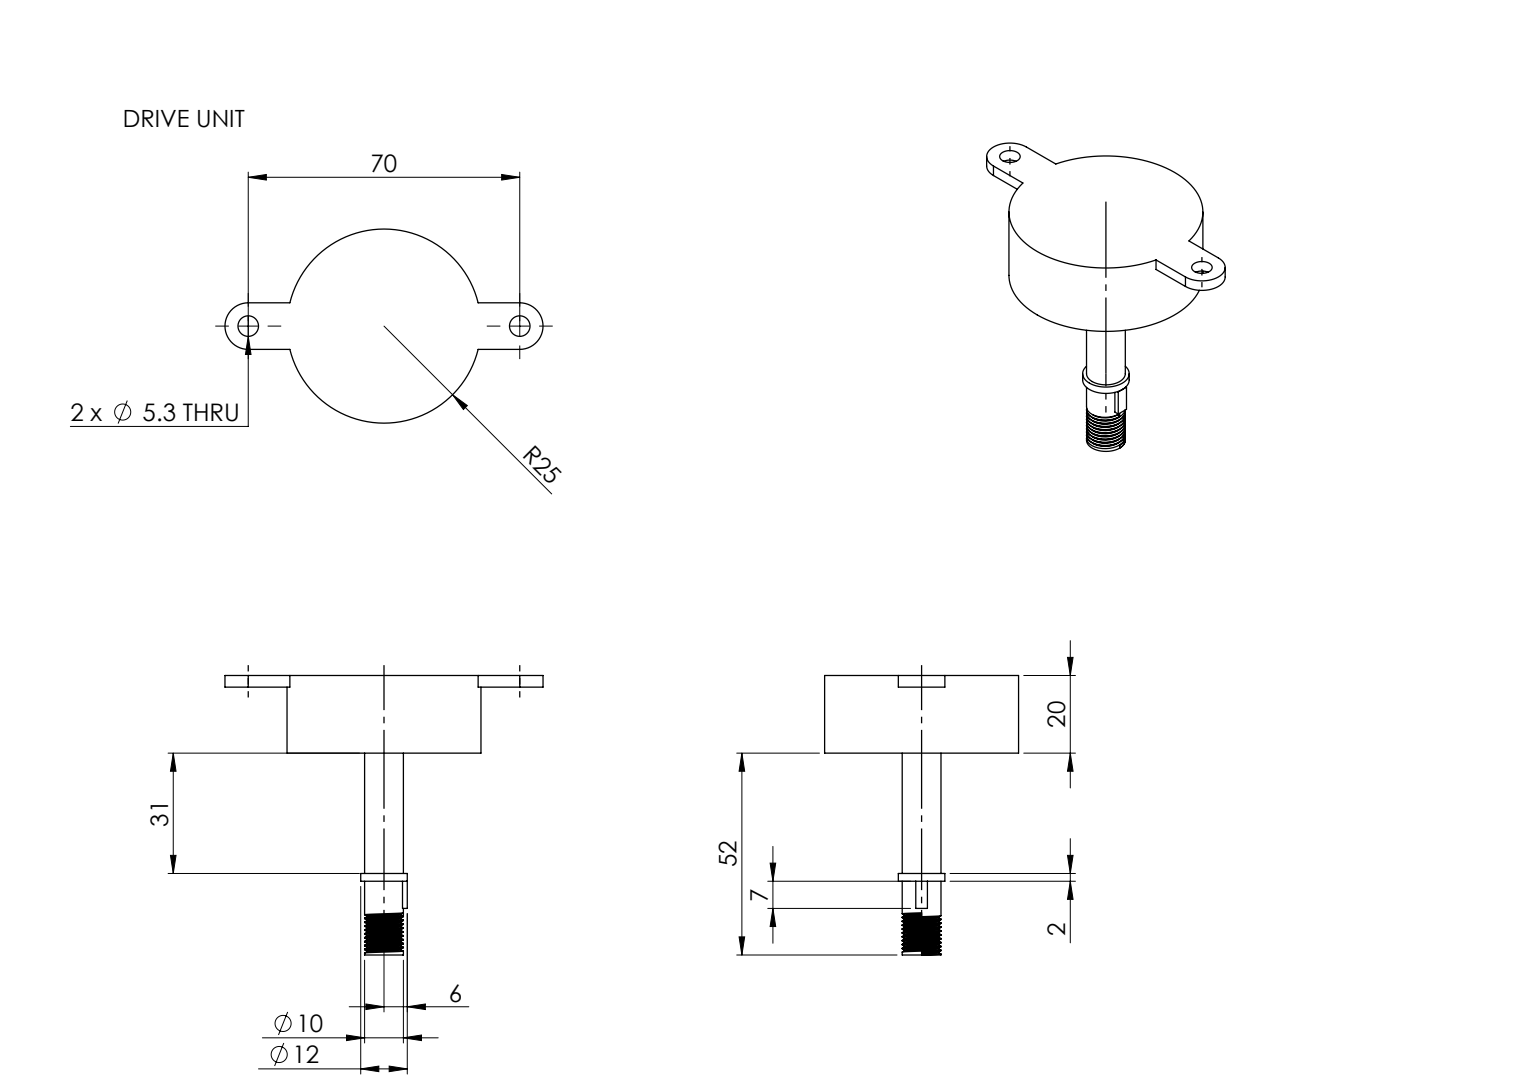
ISO-10303-21;
HEADER;
FILE_DESCRIPTION (('STEP AP214'),
    '1' );
FILE_NAME ('Drive Unit.step',
    '2026-10-08T13:56:24',
    ( '' ),
    ( '' ),
    'SwSTEP 2.0',
    'SolidWorks 2026',
    '' );
FILE_SCHEMA (( 'AUTOMOTIVE_DESIGN' ));
ENDSEC;

DATA;
#4=CARTESIAN_POINT ( 'NONE',  ( -1.846868145590737420, -24.75000000136559564, 4.458734124999999437 ) ) ;
#11=CARTESIAN_POINT ( 'NONE',  ( 1.846868145590735200, -25.50000000136559919, -4.458734125000000326 ) ) ;
#15=CARTESIAN_POINT ( 'NONE',  ( -3.535533905932738641, -28.50000000273118772, 3.535533905932737309 ) ) ;
#17=CARTESIAN_POINT ( 'NONE',  ( 3.152801135295367541, -29.31250000136559208, -3.152801135295367541 ) ) ;
#49=CARTESIAN_POINT ( 'NONE',  ( -2.071067811865478170, -24.31250000000000000, 5.000000000000000000 ) ) ;
#50=CARTESIAN_POINT ( 'NONE',  ( 5.000000000000000000, -28.18750000273119127, 2.071067811865478614 ) ) ;
#51=CARTESIAN_POINT ( 'NONE',  ( -4.458734124999999437, -26.25000000136559564, -1.846868145590735644 ) ) ;
#52=CARTESIAN_POINT ( 'NONE',  ( 3.152801135295366208, -23.56250000136559564, 3.152801135295367985 ) ) ;
#60=CARTESIAN_POINT ( 'NONE',  ( -4.458734124999999437, -23.18750000136559564, -5.460374474430324690E-16 ) ) ;
#62=CARTESIAN_POINT ( 'NONE',  ( -9.184850993605147944E-16, -30.37500000273118772, 5.000000000000000888 ) ) ;
#69=CARTESIAN_POINT ( 'NONE',  ( -3.535533905932737309, -27.62500000000000000, -3.535533905932738197 ) ) ;
#70=CARTESIAN_POINT ( 'NONE',  ( 1.846868145590736310, -28.62500000136559919, 4.458734124999999437 ) ) ;
#77=CARTESIAN_POINT ( 'NONE',  ( 2.730187237215162345E-16, -26.18750000136559564, -4.458734124999999437 ) ) ;
#79=VERTEX_POINT ( 'NONE', #13671 ) ;
#87=CARTESIAN_POINT ( 'NONE',  ( -3.535533905932738641, -30.37500000000000000, 3.535533905932737309 ) ) ;
#90=CARTESIAN_POINT ( 'NONE',  ( 3.535533905932738197, -27.00000000273118772, -3.535533905932738197 ) ) ;
#93=ORIENTED_EDGE ( 'NONE', *, *, #6840, .T. ) ;
#108=CARTESIAN_POINT ( 'NONE',  ( 5.000000000000000000, -24.06250000000000000, 2.071067811865478614 ) ) ;
#110=LINE ( 'NONE', #12615, #13102 ) ;
#113=FACE_OUTER_BOUND ( 'NONE', #15026, .T. ) ;
#122=DIRECTION ( 'NONE',  ( 0.000000000000000000, 0.000000000000000000, -1.000000000000000000 ) ) ;
#124=CARTESIAN_POINT ( 'NONE',  ( -9.184850993605147944E-16, -27.37500000273118772, 5.000000000000000000 ) ) ;
#129=CARTESIAN_POINT ( 'NONE',  ( 3.152801135295366208, -23.81250000136559564, 3.152801135295367985 ) ) ;
#130=ORIENTED_EDGE ( 'NONE', *, *, #2112, .F. ) ;
#136=EDGE_LOOP ( 'NONE', ( #1331, #8498 ) ) ;
#139=CARTESIAN_POINT ( 'NONE',  ( -1.846868145590737420, -25.00000000136559564, 4.458734124999999437 ) ) ;
#141=STYLED_ITEM ( 'NONE', ( #7237 ), #10261 ) ;
#143=PLANE ( 'NONE',  #15618 ) ;
#152=CARTESIAN_POINT ( 'NONE',  ( -1.846868145590734756, -25.12500000136559564, -4.458734125000000326 ) ) ;
#163=CARTESIAN_POINT ( 'NONE',  ( -4.458734124999999437, -25.93750000136559564, -5.460374474430324690E-16 ) ) ;
#164=ADVANCED_FACE ( 'NONE', ( #12534 ), #7474, .T. ) ;
#165=CARTESIAN_POINT ( 'NONE',  ( 0.000000000000000000, -13.00000000000000178, 0.000000000000000000 ) ) ;
#168=CARTESIAN_POINT ( 'NONE',  ( 6.123233995736766282E-16, -20.00000000000000000, -5.000000000000000000 ) ) ;
#172=CARTESIAN_POINT ( 'NONE',  ( 3.061616997868383141E-16, -30.75000000000000000, -5.000000000000000000 ) ) ;
#175=CARTESIAN_POINT ( 'NONE',  ( -3.535533905932738641, -27.50000000273118772, 3.535533905932737309 ) ) ;
#177=CARTESIAN_POINT ( 'NONE',  ( -1.846868145590734756, -31.12500000136559564, -4.458734124999999437 ) ) ;
#204=CARTESIAN_POINT ( 'NONE',  ( 1.846868145590735200, -31.25000000136559564, -4.458734125000000326 ) ) ;
#216=CARTESIAN_POINT ( 'NONE',  ( 3.061616997868383141E-16, -26.87500000273118772, -5.000000000000000000 ) ) ;
#217=CARTESIAN_POINT ( 'NONE',  ( 3.061616997868383141E-16, -27.87500000273118772, -5.000000000000000000 ) ) ;
#218=CARTESIAN_POINT ( 'NONE',  ( -1.846868145590737420, -22.00000000136559208, 4.458734124999997661 ) ) ;
#222=DIRECTION ( 'NONE',  ( -0.000000000000000000, 1.000000000000000000, -0.000000000000000000 ) ) ;
#227=EDGE_CURVE ( 'NONE', #9634, #14535, #13577, .T. ) ;
#228=ADVANCED_FACE ( 'NONE', ( #113 ), #1674, .T. ) ;
#234=CARTESIAN_POINT ( 'NONE',  ( 4.458734124999999437, -31.56250000136559564, 0.000000000000000000 ) ) ;
#240=CARTESIAN_POINT ( 'NONE',  ( 5.000000000000000000, -30.06250000000000000, 2.071067811865478614 ) ) ;
#243=CARTESIAN_POINT ( 'NONE',  ( -8.190561711645485556E-16, -26.68750000136559564, 4.458734124999999437 ) ) ;
#250=EDGE_CURVE ( 'NONE', #4014, #15267, #13743, .T. ) ;
#251=VECTOR ( 'NONE', #1802, 1000.000000000000000 ) ;
#252=CARTESIAN_POINT ( 'NONE',  ( -4.458734125000001214, -23.87500000136559564, 1.846868145590734089 ) ) ;
#257=DIRECTION ( 'NONE',  ( -0.000000000000000000, 1.000000000000000000, -0.000000000000000000 ) ) ;
#259=FACE_OUTER_BOUND ( 'NONE', #15924, .T. ) ;
#260=CARTESIAN_POINT ( 'NONE',  ( 5.000000000000000000, -29.00000000000000000, 0.000000000000000000 ) ) ;
#261=DIRECTION ( 'NONE',  ( -1.000000000000000000, 0.000000000000000000, 1.239088197126290570E-16 ) ) ;
#262=FACE_OUTER_BOUND ( 'NONE', #12296, .T. ) ;
#263=CARTESIAN_POINT ( 'NONE',  ( 2.071067811865476394, -27.31250000273118417, 5.000000000000000000 ) ) ;
#265=CARTESIAN_POINT ( 'NONE',  ( -8.190561711645485556E-16, -28.68750000136559564, 4.458734124999999437 ) ) ;
#270=ORIENTED_EDGE ( 'NONE', *, *, #4846, .T. ) ;
#274=CARTESIAN_POINT ( 'NONE',  ( 4.458734125000000326, -30.62500000136559208, -1.846868145590734978 ) ) ;
#278=( BOUNDED_CURVE ( )  B_SPLINE_CURVE ( 2, ( #14307, #13082, #15370, #11632, #13162, #12840, #4291, #11788, #15531 ),
 .UNSPECIFIED., .F., .F. ) 
 B_SPLINE_CURVE_WITH_KNOTS ( ( 3, 2, 2, 2, 3 ),
 ( 0.1750000000000001554, 0.1875000000000000833, 0.2000000000000000111, 0.2124999999999999389, 0.2249999999999998668 ),
 .UNSPECIFIED. ) 
 CURVE ( )  GEOMETRIC_REPRESENTATION_ITEM ( )  RATIONAL_B_SPLINE_CURVE ( ( 0.9999999999999990008, 0.9238795325112877377, 1.000000000000000000, 0.9238795325112867385, 1.000000000000000000, 0.9238795325112867385, 1.000000000000000000, 0.9238795325112876267, 0.9999999999999991118 ) ) 
 REPRESENTATION_ITEM ( '' )  );
#291=CARTESIAN_POINT ( 'NONE',  ( -9.184850993605147944E-16, -28.37500000273118772, 5.000000000000000000 ) ) ;
#292=EDGE_CURVE ( 'NONE', #10237, #3154, #5220, .T. ) ;
#293=CARTESIAN_POINT ( 'NONE',  ( -9.184850993605147944E-16, -21.37500000273118772, 5.000000000000000000 ) ) ;
#301=CYLINDRICAL_SURFACE ( 'NONE', #15098, 2.649999999999992806 ) ;
#305=CARTESIAN_POINT ( 'NONE',  ( -24.26932219902320043, 37.00000000000000000, -5.999999999999984901 ) ) ;
#308=ORIENTED_EDGE ( 'NONE', *, *, #7729, .F. ) ;
#311=DIRECTION ( 'NONE',  ( -0.000000000000000000, 1.000000000000000000, -0.000000000000000000 ) ) ;
#321=CARTESIAN_POINT ( 'NONE',  ( -3.152801135295367985, -22.81250000136559564, 3.152801135295367096 ) ) ;
#324=DIRECTION ( 'NONE',  ( 0.000000000000000000, 1.000000000000000000, 0.000000000000000000 ) ) ;
#328=CARTESIAN_POINT ( 'NONE',  ( 1.846868145590735200, -22.25000000136559564, -4.458734125000000326 ) ) ;
#331=CARTESIAN_POINT ( 'NONE',  ( -5.000000000000000888, -28.56250000000000000, -2.071067811865475949 ) ) ;
#335=EDGE_CURVE ( 'NONE', #10196, #14496, #7821, .T. ) ;
#336=CARTESIAN_POINT ( 'NONE',  ( -3.535533905932737309, -29.62500000000000355, -3.535533905932738197 ) ) ;
#339=CARTESIAN_POINT ( 'NONE',  ( 3.535533905932736864, -23.25000000273118772, 3.535533905932738641 ) ) ;
#341=CARTESIAN_POINT ( 'NONE',  ( -9.184850993605147944E-16, -24.37500000273118772, 5.000000000000000000 ) ) ;
#346=ORIENTED_EDGE ( 'NONE', *, *, #4980, .T. ) ;
#349=VERTEX_POINT ( 'NONE', #8867 ) ;
#351=CARTESIAN_POINT ( 'NONE',  ( -5.000000000000000000, -31.50000000000000000, -6.123233995736766282E-16 ) ) ;
#352=PLANE ( 'NONE',  #15206 ) ;
#353=VECTOR ( 'NONE', #2265, 1000.000000000000000 ) ;
#356=DIRECTION ( 'NONE',  ( 0.000000000000000000, 0.000000000000000000, 1.000000000000000000 ) ) ;
#357=ORIENTED_EDGE ( 'NONE', *, *, #14558, .T. ) ;
#365=CARTESIAN_POINT ( 'NONE',  ( 3.061616997868383043E-15, 20.00000000000000000, -25.00000000000000000 ) ) ;
#367=CARTESIAN_POINT ( 'NONE',  ( 6.123233995736766282E-16, -20.00000000000000000, -5.000000000000000000 ) ) ;
#372=CARTESIAN_POINT ( 'NONE',  ( 1.846868145590736310, -21.87500000136559208, 4.458734124999997661 ) ) ;
#376=CARTESIAN_POINT ( 'NONE',  ( -3.535533905932738641, -26.50000000273118772, 3.535533905932737309 ) ) ;
#379=VERTEX_POINT ( 'NONE', #1738 ) ;
#391=CARTESIAN_POINT ( 'NONE',  ( -4.458734125000001214, -22.87500000136559564, 1.846868145590734089 ) ) ;
#397=ORIENTED_EDGE ( 'NONE', *, *, #8592, .F. ) ;
#399=CARTESIAN_POINT ( 'NONE',  ( 3.152801135295367541, -31.56250000136559564, -3.152801135295367541 ) ) ;
#401=CARTESIAN_POINT ( 'NONE',  ( 0.000000000000000000, -32.00000000000000000, 0.000000000000000000 ) ) ;
#403=CIRCLE ( 'NONE', #1678, 25.00000000000000000 ) ;
#409=CARTESIAN_POINT ( 'NONE',  ( 5.000000000000000000, -29.06250000000000000, 2.071067811865478614 ) ) ;
#413=CARTESIAN_POINT ( 'NONE',  ( -3.535533905932738641, -24.50000000273118772, 3.535533905932737309 ) ) ;
#414=AXIS2_PLACEMENT_3D ( 'NONE', #3644, #8589, #5995 ) ;
#416=CARTESIAN_POINT ( 'NONE',  ( 4.458734124999999437, -26.37500000136559564, -1.846868145590734978 ) ) ;
#417=CARTESIAN_POINT ( 'NONE',  ( -35.00000000000000000, 40.00000000000000000, 0.000000000000000000 ) ) ;
#422=ADVANCED_FACE ( 'NONE', ( #15007 ), #3921, .T. ) ;
#426=CIRCLE ( 'NONE', #9451, 2.649999999999985700 ) ;
#428=CARTESIAN_POINT ( 'NONE',  ( 1.846868145590735200, -30.50000000136559919, -4.458734125000000326 ) ) ;
#432=CARTESIAN_POINT ( 'NONE',  ( 4.729367062499999719, -31.84375000068279959, 0.000000000000000000 ) ) ;
#436=CARTESIAN_POINT ( 'NONE',  ( -4.458734124999999437, -30.93750000136559564, -5.460374474430324690E-16 ) ) ;
#445=CARTESIAN_POINT ( 'NONE',  ( -3.535533905932737309, -28.75000000273118772, -3.535533905932738197 ) ) ;
#446=EDGE_CURVE ( 'NONE', #12836, #3368, #3237, .T. ) ;
#453=CARTESIAN_POINT ( 'NONE',  ( 3.152801135295367541, -23.56250000136559564, -3.152801135295367541 ) ) ;
#455=FACE_BOUND ( 'NONE', #11569, .T. ) ;
#464=( BOUNDED_CURVE ( )  B_SPLINE_CURVE ( 2, ( #5096, #12595, #1539, #6477, #12273, #177, #13559, #9939, #5254, #10191, #8585, #11390, #3640, #13806, #11315, #2658, #13474, #3714, #1368, #10032, #8661, #14967, #11084, #13650, #3882, #14877, #8901, #7611, #2741, #2411, #2579, #6158, #7531, #7454, #17, #4935, #12359, #12432, #15041, #1291, #8824, #12510, #6236, #11152, #265, #13725, #1451, #5010, #15363, #6792, #8985, #12990, #6636, #5424, #14147, #9068, #4372, #6553, #3076, #5661, #1695, #15207, #1612, #15451, #1927, #4120, #11550, #4034, #6877, #13898, #11468, #10427, #14227, #5497, #576, #7936, #12915, #7853, #11782, #4285, #12670, #416, #15113, #9305, #10278, #2826, #736, #7780, #4197, #11626, #3151, #9223, #8096, #8018, #11700, #1849, #504, #9144, #5339, #13970, #2902, #12750, #2984, #10356, #15283, #14057, #12833, #1777, #655, #5581, #6725, #10517, #810, #8263, #7406, #13156, #5730, #5809, #14834, #8701, #6110, #13603, #2090, #887, #9821, #4518, #52, #2013, #14750, #1328, #7035, #11935, #7323, #12310, #3600, #9453, #12227, #10665, #1249, #7489, #15600, #11037, #9895, #1166, #11027, #8547, #8620, #3311, #12392, #4896, #8175, #10601, #2451, #13435, #6197, #10745, #15525, #4968, #11114, #15681, #4441 ),
 .UNSPECIFIED., .F., .F. ) 
 B_SPLINE_CURVE_WITH_KNOTS ( ( 3, 2, 2, 2, 2, 2, 2, 2, 2, 2, 2, 2, 2, 2, 2, 2, 2, 2, 2, 2, 2, 2, 2, 2, 2, 2, 2, 2, 2, 2, 2, 2, 2, 2, 2, 2, 2, 2, 2, 2, 2, 2, 2, 2, 2, 2, 2, 2, 2, 2, 2, 2, 2, 2, 2, 2, 2, 2, 2, 2, 2, 2, 2, 2, 2, 2, 2, 2, 2, 2, 2, 2, 2, 2, 2, 2, 2, 2, 2, 2, 3 ),
 ( 0.000000000000000000, 0.01250000000000000069, 0.02500000000000000139, 0.03749999999999999861, 0.05000000000000000278, 0.06250000000000000000, 0.07499999999999999722, 0.08749999999999999445, 0.1000000000000000056, 0.1125000000000000028, 0.1250000000000000000, 0.1375000000000000111, 0.1499999999999999944, 0.1625000000000000056, 0.1749999999999999889, 0.1875000000000000000, 0.2000000000000000111, 0.2124999999999999944, 0.2250000000000000056, 0.2374999999999999889, 0.2500000000000000000, 0.2625000000000000111, 0.2750000000000000222, 0.2874999999999999778, 0.2999999999999999889, 0.3125000000000000000, 0.3250000000000000111, 0.3375000000000000222, 0.3499999999999999778, 0.3624999999999999889, 0.3750000000000000000, 0.3875000000000000111, 0.4000000000000000222, 0.4124999999999999778, 0.4249999999999999889, 0.4375000000000000000, 0.4500000000000000111, 0.4625000000000000222, 0.4749999999999999778, 0.4874999999999999889, 0.5000000000000000000, 0.5124999999999999556, 0.5250000000000000222, 0.5374999999999999778, 0.5500000000000000444, 0.5625000000000000000, 0.5749999999999999556, 0.5875000000000000222, 0.5999999999999999778, 0.6125000000000000444, 0.6250000000000000000, 0.6374999999999999556, 0.6500000000000000222, 0.6624999999999999778, 0.6750000000000000444, 0.6875000000000000000, 0.6999999999999999556, 0.7125000000000000222, 0.7249999999999999778, 0.7375000000000000444, 0.7500000000000000000, 0.7624999999999999556, 0.7750000000000000222, 0.7874999999999999778, 0.8000000000000000444, 0.8125000000000000000, 0.8249999999999999556, 0.8375000000000000222, 0.8499999999999999778, 0.8625000000000000444, 0.8750000000000000000, 0.8874999999999999556, 0.9000000000000000222, 0.9124999999999999778, 0.9250000000000000444, 0.9375000000000000000, 0.9499999999999999556, 0.9625000000000000222, 0.9749999999999999778, 0.9875000000000000444, 1.000000000000000000 ),
 .UNSPECIFIED. ) 
 CURVE ( )  GEOMETRIC_REPRESENTATION_ITEM ( )  RATIONAL_B_SPLINE_CURVE ( ( 1.000000000000000000, 0.9238795325112867385, 1.000000000000000000, 0.9238795325112867385, 1.000000000000000000, 0.9238795325112867385, 1.000000000000000000, 0.9238795325112867385, 1.000000000000000000, 0.9238795325112867385, 1.000000000000000000, 0.9238795325112867385, 1.000000000000000000, 0.9238795325112867385, 1.000000000000000000, 0.9238795325112867385, 1.000000000000000000, 0.9238795325112867385, 1.000000000000000000, 0.9238795325112867385, 1.000000000000000000, 0.9238795325112867385, 1.000000000000000000, 0.9238795325112867385, 1.000000000000000000, 0.9238795325112867385, 1.000000000000000000, 0.9238795325112867385, 1.000000000000000000, 0.9238795325112867385, 1.000000000000000000, 0.9238795325112867385, 1.000000000000000000, 0.9238795325112867385, 1.000000000000000000, 0.9238795325112867385, 1.000000000000000000, 0.9238795325112867385, 1.000000000000000000, 0.9238795325112867385, 1.000000000000000000, 0.9238795325112867385, 1.000000000000000000, 0.9238795325112867385, 1.000000000000000000, 0.9238795325112867385, 1.000000000000000000, 0.9238795325112867385, 1.000000000000000000, 0.9238795325112867385, 1.000000000000000000, 0.9238795325112867385, 1.000000000000000000, 0.9238795325112867385, 1.000000000000000000, 0.9238795325112867385, 1.000000000000000000, 0.9238795325112867385, 1.000000000000000000, 0.9238795325112867385, 1.000000000000000000, 0.9238795325112867385, 1.000000000000000000, 0.9238795325112867385, 1.000000000000000000, 0.9238795325112867385, 1.000000000000000000, 0.9238795325112867385, 1.000000000000000000, 0.9238795325112867385, 1.000000000000000000, 0.9238795325112867385, 1.000000000000000000, 0.9238795325112867385, 1.000000000000000000, 0.9238795325112867385, 1.000000000000000000, 0.9238795325112867385, 1.000000000000000000, 0.9238795325112867385, 1.000000000000000000, 0.9238795325112867385, 1.000000000000000000, 0.9238795325112867385, 1.000000000000000000, 0.9238795325112867385, 1.000000000000000000, 0.9238795325112867385, 1.000000000000000000, 0.9238795325112867385, 1.000000000000000000, 0.9238795325112867385, 1.000000000000000000, 0.9238795325112867385, 1.000000000000000000, 0.9238795325112867385, 1.000000000000000000, 0.9238795325112867385, 1.000000000000000000, 0.9238795325112867385, 1.000000000000000000, 0.9238795325112867385, 1.000000000000000000, 0.9238795325112867385, 1.000000000000000000, 0.9238795325112867385, 1.000000000000000000, 0.9238795325112867385, 1.000000000000000000, 0.9238795325112867385, 1.000000000000000000, 0.9238795325112867385, 1.000000000000000000, 0.9238795325112867385, 1.000000000000000000, 0.9238795325112867385, 1.000000000000000000, 0.9238795325112867385, 1.000000000000000000, 0.9238795325112867385, 1.000000000000000000, 0.9238795325112867385, 1.000000000000000000, 0.9238795325112867385, 1.000000000000000000, 0.9238795325112867385, 1.000000000000000000, 0.9238795325112867385, 1.000000000000000000, 0.9238795325112867385, 1.000000000000000000, 0.9238795325112867385, 1.000000000000000000, 0.9238795325112867385, 1.000000000000000000, 0.9238795325112867385, 1.000000000000000000, 0.9238795325112867385, 1.000000000000000000, 0.9238795325112867385, 1.000000000000000000, 0.9238795325112867385, 1.000000000000000000, 0.9238795325112867385, 1.000000000000000000, 0.9238795325112867385, 1.000000000000000000, 0.9238795325112867385, 1.000000000000000000, 0.9238795325112867385, 1.000000000000000000, 0.9238795325112867385, 1.000000000000000000, 0.9238795325112867385, 1.000000000000000000, 0.9238795325112867385, 1.000000000000000000, 0.9238795325112867385, 1.000000000000000000, 0.9238795325112867385, 1.000000000000000000 ) ) 
 REPRESENTATION_ITEM ( '' )  );
#469=FACE_OUTER_BOUND ( 'NONE', #10752, .T. ) ;
#476=CARTESIAN_POINT ( 'NONE',  ( 1.846868145590735200, -24.25000000136559564, -4.458734125000000326 ) ) ;
#479=UNCERTAINTY_MEASURE_WITH_UNIT (LENGTH_MEASURE( 1.000000000000000082E-05 ), #11657, 'distance_accuracy_value', 'NONE');
#481=DIRECTION ( 'NONE',  ( 0.000000000000000000, 0.000000000000000000, 1.000000000000000000 ) ) ;
#483=ORIENTED_EDGE ( 'NONE', *, *, #15732, .F. ) ;
#484=ORIENTED_EDGE ( 'NONE', *, *, #9626, .T. ) ;
#485=CARTESIAN_POINT ( 'NONE',  ( 1.846868145590736310, -21.62500000136559564, 4.458734124999999437 ) ) ;
#488=DIRECTION ( 'NONE',  ( 0.000000000000000000, -0.000000000000000000, 1.000000000000000000 ) ) ;
#491=DIRECTION ( 'NONE',  ( 0.000000000000000000, 1.000000000000000000, 0.000000000000000000 ) ) ;
#494=CARTESIAN_POINT ( 'NONE',  ( 2.071067811865476394, -26.18750000000000355, 5.000000000000000000 ) ) ;
#499=EDGE_CURVE ( 'NONE', #2433, #13770, #15943, .T. ) ;
#500=CARTESIAN_POINT ( 'NONE',  ( -2.071067811865475061, -24.81250000273118417, -5.000000000000000888 ) ) ;
#503=CIRCLE ( 'NONE', #4355, 5.000000000000000000 ) ;
#504=CARTESIAN_POINT ( 'NONE',  ( 4.458734124999999437, -25.43750000136559564, 0.000000000000000000 ) ) ;
#517=DIRECTION ( 'NONE',  ( 1.000000000000000000, -0.000000000000000000, -1.239088197126290570E-16 ) ) ;
#521=EDGE_CURVE ( 'NONE', #13476, #13669, #12188, .T. ) ;
#528=CARTESIAN_POINT ( 'NONE',  ( -4.458734125000001214, -27.87500000136559564, 1.846868145590734089 ) ) ;
#529=ORIENTED_EDGE ( 'NONE', *, *, #6898, .T. ) ;
#538=CARTESIAN_POINT ( 'NONE',  ( -4.458734124999999437, -23.18750000136559564, -5.460374474430324690E-16 ) ) ;
#539=ORIENTED_EDGE ( 'NONE', *, *, #227, .F. ) ;
#548=CARTESIAN_POINT ( 'NONE',  ( 0.000000000000000000, -20.00000000000000000, 0.000000000000000000 ) ) ;
#552=CARTESIAN_POINT ( 'NONE',  ( 5.000000000000000000, -23.06250000000000000, 2.071067811865478614 ) ) ;
#555=CARTESIAN_POINT ( 'NONE',  ( 5.000000000000000888, -25.06250000273118417, -2.071067811865475505 ) ) ;
#556=FACE_OUTER_BOUND ( 'NONE', #7798, .T. ) ;
#562=CARTESIAN_POINT ( 'NONE',  ( 1.846868145590736310, -30.87500000136559564, 4.458734124999999437 ) ) ;
#570=CARTESIAN_POINT ( 'NONE',  ( -5.000000000000000000, -27.50000000000000000, -6.123233995736766282E-16 ) ) ;
#574=CARTESIAN_POINT ( 'NONE',  ( 5.000000000000000000, -23.18750000273119127, 2.071067811865478614 ) ) ;
#576=CARTESIAN_POINT ( 'NONE',  ( -3.152801135295367985, -26.81250000136559564, 3.152801135295367096 ) ) ;
#580=VERTEX_POINT ( 'NONE', #7452 ) ;
#583=ORIENTED_EDGE ( 'NONE', *, *, #907, .F. ) ;
#588=CARTESIAN_POINT ( 'NONE',  ( -3.152801135295367985, -26.06250000136559919, 3.152801135295367096 ) ) ;
#594=EDGE_LOOP ( 'NONE', ( #1579, #15115, #2346, #7475 ) ) ;
#601=EDGE_CURVE ( 'NONE', #3228, #2810, #2578, .T. ) ;
#603=DIRECTION ( 'NONE',  ( -1.000000000000000000, 0.000000000000000000, 1.239088197126290570E-16 ) ) ;
#607=UNCERTAINTY_MEASURE_WITH_UNIT (LENGTH_MEASURE( 1.000000000000000082E-05 ), #5032, 'distance_accuracy_value', 'NONE');
#611=VECTOR ( 'NONE', #13383, 1000.000000000000000 ) ;
#614=CARTESIAN_POINT ( 'NONE',  ( 3.061616997868383141E-16, -24.75000000000000000, -5.000000000000000000 ) ) ;
#627=CARTESIAN_POINT ( 'NONE',  ( 5.000000000000000888, -26.06250000273118417, -2.071067811865475505 ) ) ;
#633=CARTESIAN_POINT ( 'NONE',  ( -3.152801135295367985, -21.81250000136559208, 3.152801135295367096 ) ) ;
#639=CARTESIAN_POINT ( 'NONE',  ( -4.458734125000000326, -22.00000000136559208, -1.846868145590735644 ) ) ;
#649=CARTESIAN_POINT ( 'NONE',  ( 5.000000000000000888, -27.93750000000000711, -2.071067811865475505 ) ) ;
#653=CARTESIAN_POINT ( 'NONE',  ( -9.184850993605147944E-16, -23.37500000273118772, 5.000000000000000000 ) ) ;
#654=ORIENTED_EDGE ( 'NONE', *, *, #7999, .T. ) ;
#655=CARTESIAN_POINT ( 'NONE',  ( -8.190561711645485556E-16, -24.68750000136559564, 4.458734124999999437 ) ) ;
#661=CARTESIAN_POINT ( 'NONE',  ( 4.769696007084728073, -20.00000000000000000, 1.500000000000000000 ) ) ;
#666=CARTESIAN_POINT ( 'NONE',  ( 3.152801135295367541, -26.56250000136559564, -3.152801135295367541 ) ) ;
#680=DIRECTION ( 'NONE',  ( -0.000000000000000000, -1.000000000000000000, -0.000000000000000000 ) ) ;
#689=EDGE_LOOP ( 'NONE', ( #8517, #6406, #1835, #397 ) ) ;
#693=CARTESIAN_POINT ( 'NONE',  ( 3.535533905932736864, -27.12500000000000000, 3.535533905932738641 ) ) ;
#695=ORIENTED_EDGE ( 'NONE', *, *, #15597, .F. ) ;
#704=CARTESIAN_POINT ( 'NONE',  ( -5.000000000000000000, -25.50000000000000355, -6.123233995736766282E-16 ) ) ;
#711=CARTESIAN_POINT ( 'NONE',  ( -4.458734124999999437, -28.25000000136559919, -1.846868145590735644 ) ) ;
#713=EDGE_CURVE ( 'NONE', #79, #15920, #10355, .T. ) ;
#719=CARTESIAN_POINT ( 'NONE',  ( -4.458734125000000326, -28.25000000136559208, -1.846868145590735644 ) ) ;
#720=CARTESIAN_POINT ( 'NONE',  ( 6.123233995736766282E-16, -20.00000000000000000, -5.000000000000000000 ) ) ;
#721=VECTOR ( 'NONE', #9973, 1000.000000000000114 ) ;
#727=DIRECTION ( 'NONE',  ( -0.000000000000000000, -1.000000000000000000, -0.000000000000000000 ) ) ;
#728=CARTESIAN_POINT ( 'NONE',  ( 5.000000000000000000, -24.00000000000000000, 0.000000000000000000 ) ) ;
#733=CARTESIAN_POINT ( 'NONE',  ( 5.000000000000000000, -21.18750000273119127, 2.071067811865478614 ) ) ;
#735=ORIENTED_EDGE ( 'NONE', *, *, #13938, .F. ) ;
#736=CARTESIAN_POINT ( 'NONE',  ( -3.152801135295367096, -26.06250000136559564, -3.152801135295367541 ) ) ;
#741=AXIS2_PLACEMENT_3D ( 'NONE', #14902, #12451, #7471 ) ;
#747=CARTESIAN_POINT ( 'NONE',  ( -1.846868145590734756, -29.37500000136559564, -4.458734125000000326 ) ) ;
#755=ORIENTED_EDGE ( 'NONE', *, *, #9626, .F. ) ;
#774=CARTESIAN_POINT ( 'NONE',  ( 5.000000000000000000, -27.00000000000000000, 0.000000000000000000 ) ) ;
#776=ORIENTED_EDGE ( 'NONE', *, *, #7729, .T. ) ;
#787=CARTESIAN_POINT ( 'NONE',  ( 3.061616997868383141E-16, -24.87500000273118417, -5.000000000000000000 ) ) ;
#788=CARTESIAN_POINT ( 'NONE',  ( 4.458734124999999437, -28.62500000136559564, -1.846868145590734978 ) ) ;
#796=CARTESIAN_POINT ( 'NONE',  ( 3.152801135295366208, -25.81250000136559564, 3.152801135295367985 ) ) ;
#804=CARTESIAN_POINT ( 'NONE',  ( -3.535533905932738641, -26.37500000000000355, 3.535533905932737309 ) ) ;
#808=CARTESIAN_POINT ( 'NONE',  ( -3.152801135295367096, -29.06250000136559564, -3.152801135295367541 ) ) ;
#809=ORIENTED_EDGE ( 'NONE', *, *, #11477, .T. ) ;
#810=CARTESIAN_POINT ( 'NONE',  ( 4.458734124999999437, -24.43750000136559564, 0.000000000000000000 ) ) ;
#813=ORIENTED_EDGE ( 'NONE', *, *, #12222, .F. ) ;
#815=CARTESIAN_POINT ( 'NONE',  ( -3.152801135295367096, -28.06250000136559564, -3.152801135295367541 ) ) ;
#818=CARTESIAN_POINT ( 'NONE',  ( -3.535533905932738641, -24.50000000273118772, 3.535533905932737309 ) ) ;
#821=CARTESIAN_POINT ( 'NONE',  ( -3.152801135295367096, -26.31250000136559564, -3.152801135295367541 ) ) ;
#822=DIRECTION ( 'NONE',  ( -1.000000000000000000, 0.000000000000000000, 1.239088197126290570E-16 ) ) ;
#829=EDGE_LOOP ( 'NONE', ( #13631, #3584, #12937, #6136 ) ) ;
#831=ORIENTED_EDGE ( 'NONE', *, *, #10965, .F. ) ;
#836=CARTESIAN_POINT ( 'NONE',  ( 3.061616997868383141E-16, -27.75000000000000000, -5.000000000000000000 ) ) ;
#846=EDGE_CURVE ( 'NONE', #8138, #15819, #13214, .T. ) ;
#851=EDGE_LOOP ( 'NONE', ( #9621, #3536, #2832, #14469 ) ) ;
#856=LINE ( 'NONE', #14435, #15169 ) ;
#858=CYLINDRICAL_SURFACE ( 'NONE', #8255, 5.000000000000000000 ) ;
#863=CARTESIAN_POINT ( 'NONE',  ( 1.846868145590736310, -27.87500000136559564, 4.458734124999997661 ) ) ;
#870=ADVANCED_FACE ( 'NONE', ( #1789 ), #9154, .T. ) ;
#875=CARTESIAN_POINT ( 'NONE',  ( 1.846868145590735200, -25.50000000136559919, -4.458734125000000326 ) ) ;
#880=( BOUNDED_CURVE ( )  B_SPLINE_CURVE ( 2, ( #1973, #6919, #693, #11825, #774, #5696, #10633, #15564, #1149 ),
 .UNSPECIFIED., .F., .F. ) 
 B_SPLINE_CURVE_WITH_KNOTS ( ( 3, 2, 2, 2, 3 ),
 ( 0.4750000000000000888, 0.4875000000000000999, 0.5000000000000001110, 0.5125000000000000666, 0.5250000000000001332 ),
 .UNSPECIFIED. ) 
 CURVE ( )  GEOMETRIC_REPRESENTATION_ITEM ( )  RATIONAL_B_SPLINE_CURVE ( ( 0.9999999999999993339, 0.9238795325112874046, 1.000000000000000000, 0.9238795325112867385, 1.000000000000000000, 0.9238795325112867385, 1.000000000000000000, 0.9238795325112860723, 1.000000000000000666 ) ) 
 REPRESENTATION_ITEM ( '' )  );
#885=CARTESIAN_POINT ( 'NONE',  ( 1.846868145590736310, -29.62500000136559208, 4.458734124999999437 ) ) ;
#887=CARTESIAN_POINT ( 'NONE',  ( -1.846868145590737420, -23.75000000136559564, 4.458734124999997661 ) ) ;
#895=CARTESIAN_POINT ( 'NONE',  ( -4.458734124999999437, -29.93750000136559564, -5.460374474430324690E-16 ) ) ;
#898=CARTESIAN_POINT ( 'NONE',  ( -5.000000000000000888, -24.56250000273118772, 2.071067811865474617 ) ) ;
#899=FACE_OUTER_BOUND ( 'NONE', #14701, .T. ) ;
#901=CARTESIAN_POINT ( 'NONE',  ( -8.190561711645485556E-16, -28.93750000136559564, 4.458734124999999437 ) ) ;
#907=EDGE_CURVE ( 'NONE', #8217, #4663, #4887, .T. ) ;
#909=ORIENTED_EDGE ( 'NONE', *, *, #7781, .F. ) ;
#926=AXIS2_PLACEMENT_3D ( 'NONE', #14707, #3629, #488 ) ;
#929=CARTESIAN_POINT ( 'NONE',  ( 6.000000000000000000, -13.00000000000000178, 1.500000000000000000 ) ) ;
#933=CIRCLE ( 'NONE', #2729, 5.000000000000000000 ) ;
#936=DIRECTION ( 'NONE',  ( 0.000000000000000000, 0.000000000000000000, -1.000000000000000000 ) ) ;
#940=CARTESIAN_POINT ( 'NONE',  ( -8.190561711645485556E-16, -30.93750000136559564, 4.458734124999999437 ) ) ;
#943=AXIS2_PLACEMENT_3D ( 'NONE', #9492, #14262, #5694 ) ;
#949=AXIS2_PLACEMENT_3D ( 'NONE', #12692, #12456, #11172 ) ;
#950=CARTESIAN_POINT ( 'NONE',  ( -8.190561711645485556E-16, -26.93750000136559564, 4.458734124999999437 ) ) ;
#951=DIRECTION ( 'NONE',  ( 0.000000000000000000, 0.000000000000000000, 1.000000000000000000 ) ) ;
#959=CARTESIAN_POINT ( 'NONE',  ( 5.000000000000000000, -23.06250000000000000, 2.071067811865478614 ) ) ;
#961=CARTESIAN_POINT ( 'NONE',  ( -5.000000000000000000, -21.62500000273118772, -6.123233995736766282E-16 ) ) ;
#962=CARTESIAN_POINT ( 'NONE',  ( 3.061616997868383141E-16, -27.75000000000000000, -5.000000000000000000 ) ) ;
#963=CARTESIAN_POINT ( 'NONE',  ( -9.184850993605147944E-16, -22.37500000273118417, 5.000000000000000000 ) ) ;
#970=CARTESIAN_POINT ( 'NONE',  ( -8.190561711645485556E-16, -28.68750000136559564, 4.458734124999999437 ) ) ;
#973=CARTESIAN_POINT ( 'NONE',  ( -2.071067811865492381, -24.43750000273118772, 4.999999999999985789 ) ) ;
#974=( BOUNDED_CURVE ( )  B_SPLINE_CURVE ( 2, ( #5596, #5515, #12932, #4387, #6567 ),
 .UNSPECIFIED., .F., .F. ) 
 B_SPLINE_CURVE_WITH_KNOTS ( ( 3, 2, 3 ),
 ( 0.000000000000000000, 0.01250000000000001110, 0.02500000000000002220 ),
 .UNSPECIFIED. ) 
 CURVE ( )  GEOMETRIC_REPRESENTATION_ITEM ( )  RATIONAL_B_SPLINE_CURVE ( ( 1.000000000000000000, 0.9238795325112867385, 1.000000000000000000, 0.9238795325112866275, 1.000000000000000222 ) ) 
 REPRESENTATION_ITEM ( '' )  );
#980=CARTESIAN_POINT ( 'NONE',  ( -1.846868145590734756, -23.37500000136559564, -4.458734125000000326 ) ) ;
#983=CARTESIAN_POINT ( 'NONE',  ( -2.071067811865475061, -30.81250000273118772, -5.000000000000000888 ) ) ;
#985=ORIENTED_EDGE ( 'NONE', *, *, #11874, .T. ) ;
#990=AXIS2_PLACEMENT_3D ( 'NONE', #10557, #15485, #3024 ) ;
#1004=ORIENTED_EDGE ( 'NONE', *, *, #13938, .T. ) ;
#1006=EDGE_LOOP ( 'NONE', ( #7439, #10537, #3336, #10117, #9918, #9746, #14886, #3496 ) ) ;
#1017=DIRECTION ( 'NONE',  ( 0.000000000000000000, 1.000000000000000000, 0.000000000000000000 ) ) ;
#1018=CARTESIAN_POINT ( 'NONE',  ( -3.152801135295367985, -29.06250000136559564, 3.152801135295367096 ) ) ;
#1026=CARTESIAN_POINT ( 'NONE',  ( -1.846868145590734756, -23.37500000136559564, -4.458734125000000326 ) ) ;
#1027=CARTESIAN_POINT ( 'NONE',  ( -35.00000000000000000, 37.00000000000000000, 0.000000000000000000 ) ) ;
#1035=CARTESIAN_POINT ( 'NONE',  ( 5.000000000000000888, -22.06250000273119127, -2.071067811865475505 ) ) ;
#1042=CARTESIAN_POINT ( 'NONE',  ( -3.152801135295367096, -29.06250000136559564, -3.152801135295367541 ) ) ;
#1043=EDGE_CURVE ( 'NONE', #8138, #8374, #4686, .T. ) ;
#1050=CARTESIAN_POINT ( 'NONE',  ( -1.846868145590734756, -22.37500000136559564, -4.458734125000000326 ) ) ;
#1053=CARTESIAN_POINT ( 'NONE',  ( -5.000000000000000888, -30.68750000273118772, -2.071067811865475949 ) ) ;
#1073=ORIENTED_EDGE ( 'NONE', *, *, #9578, .F. ) ;
#1086=CARTESIAN_POINT ( 'NONE',  ( -5.000000000000000000, -24.50000000000000000, -6.123233995736766282E-16 ) ) ;
#1088=CARTESIAN_POINT ( 'NONE',  ( 3.152801135295367541, -26.56250000136559564, -3.152801135295367541 ) ) ;
#1096=CARTESIAN_POINT ( 'NONE',  ( -3.152801135295367096, -23.31250000136559564, -3.152801135295367541 ) ) ;
#1097=DIRECTION ( 'NONE',  ( -0.000000000000000000, -1.000000000000000000, -0.000000000000000000 ) ) ;
#1100=DIRECTION ( 'NONE',  ( 0.000000000000000000, -1.000000000000000000, 0.000000000000000000 ) ) ;
#1102=CARTESIAN_POINT ( 'NONE',  ( 3.061616997868383141E-16, -23.75000000000000000, -5.000000000000000000 ) ) ;
#1105=LINE ( 'NONE', #10970, #4851 ) ;
#1106=CARTESIAN_POINT ( 'NONE',  ( -4.458734124999999437, -26.93750000136559564, -5.460374474430324690E-16 ) ) ;
#1108=VERTEX_POINT ( 'NONE', #2026 ) ;
#1111=ORIENTED_EDGE ( 'NONE', *, *, #5804, .F. ) ;
#1115=CARTESIAN_POINT ( 'NONE',  ( -4.458734125000001214, -24.87500000136559919, 1.846868145590734089 ) ) ;
#1123=CARTESIAN_POINT ( 'NONE',  ( -3.152801135295367096, -25.31250000136559564, -3.152801135295367541 ) ) ;
#1139=FACE_OUTER_BOUND ( 'NONE', #10434, .T. ) ;
#1140=EDGE_CURVE ( 'NONE', #4136, #11992, #9616, .T. ) ;
#1141=CARTESIAN_POINT ( 'NONE',  ( 3.535533905932738197, -27.87500000000000000, -3.535533905932738197 ) ) ;
#1149=CARTESIAN_POINT ( 'NONE',  ( 3.061616997868383141E-16, -26.75000000000000000, -5.000000000000000000 ) ) ;
#1162=CARTESIAN_POINT ( 'NONE',  ( -5.000000000000000888, -29.68750000273118417, -2.071067811865475949 ) ) ;
#1165=CARTESIAN_POINT ( 'NONE',  ( -8.190561711645485556E-16, -25.93750000136559564, 4.458734124999999437 ) ) ;
#1166=CARTESIAN_POINT ( 'NONE',  ( 4.458734124999997661, -22.50000000136559564, 1.846868145590737864 ) ) ;
#1172=ORIENTED_EDGE ( 'NONE', *, *, #6097, .F. ) ;
#1173=CARTESIAN_POINT ( 'NONE',  ( -3.152801135295367985, -25.06250000136559564, 3.152801135295367096 ) ) ;
#1174=CARTESIAN_POINT ( 'NONE',  ( -5.000000000000000000, -23.62500000273118772, -6.123233995736766282E-16 ) ) ;
#1177=CARTESIAN_POINT ( 'NONE',  ( 35.00000000000000000, 37.00000000000000000, 5.999999999999991118 ) ) ;
#1179=EDGE_CURVE ( 'NONE', #12690, #11826, #3166, .T. ) ;
#1187=CARTESIAN_POINT ( 'NONE',  ( 4.458734125000000326, -26.37500000136559564, -1.846868145590734978 ) ) ;
#1195=DIRECTION ( 'NONE',  ( -1.000000000000000000, 0.000000000000000000, -0.000000000000000000 ) ) ;
#1196=CARTESIAN_POINT ( 'NONE',  ( -1.846868145590737420, -23.75000000136559208, 4.458734124999999437 ) ) ;
#1204=CARTESIAN_POINT ( 'NONE',  ( 6.000000000000000000, -20.00000000000000000, 1.500000000000000000 ) ) ;
#1207=CARTESIAN_POINT ( 'NONE',  ( 2.730187237215162345E-16, -25.43750000136559564, -4.458734124999999437 ) ) ;
#1211=CARTESIAN_POINT ( 'NONE',  ( -5.000000000000000888, -28.68750000273119127, -2.071067811865475949 ) ) ;
#1219=CIRCLE ( 'NONE', #5862, 5.000000000000000000 ) ;
#1237=FACE_OUTER_BOUND ( 'NONE', #12435, .T. ) ;
#1243=CARTESIAN_POINT ( 'NONE',  ( 5.000000000000000000, -27.18750000273119127, 2.071067811865478614 ) ) ;
#1248=CARTESIAN_POINT ( 'NONE',  ( -1.846868145590734756, -27.37500000136559564, -4.458734124999999437 ) ) ;
#1249=CARTESIAN_POINT ( 'NONE',  ( -3.152801135295367985, -22.81250000136559564, 3.152801135295367096 ) ) ;
#1258=CARTESIAN_POINT ( 'NONE',  ( -8.190561711645485556E-16, -21.93750000136559208, 4.458734124999999437 ) ) ;
#1264=LINE ( 'NONE', #1177, #4309 ) ;
#1266=CIRCLE ( 'NONE', #10326, 5.000000000000000000 ) ;
#1270=CARTESIAN_POINT ( 'NONE',  ( 3.152801135295367541, -26.31250000136559564, -3.152801135295367541 ) ) ;
#1277=CARTESIAN_POINT ( 'NONE',  ( 1.846868145590735200, -25.25000000136559564, -4.458734125000000326 ) ) ;
#1286=CARTESIAN_POINT ( 'NONE',  ( 1.846868145590735200, -24.50000000136559564, -4.458734125000000326 ) ) ;
#1289=CARTESIAN_POINT ( 'NONE',  ( 3.535533905932738197, -28.00000000273118772, -3.535533905932738197 ) ) ;
#1291=CARTESIAN_POINT ( 'NONE',  ( -4.458734124999999437, -29.00000000136559564, -1.846868145590735644 ) ) ;
#1294=( BOUNDED_CURVE ( )  B_SPLINE_CURVE ( 2, ( #15589, #13146, #12302, #14666, #6099, #4506, #9443, #12144, #3592 ),
 .UNSPECIFIED., .F., .F. ) 
 B_SPLINE_CURVE_WITH_KNOTS ( ( 3, 2, 2, 2, 3 ),
 ( 0.2250000000000001998, 0.2375000000000000999, 0.2500000000000000555, 0.2624999999999999556, 0.2749999999999999112 ),
 .UNSPECIFIED. ) 
 CURVE ( )  GEOMETRIC_REPRESENTATION_ITEM ( )  RATIONAL_B_SPLINE_CURVE ( ( 0.9999999999999987788, 0.9238795325112879597, 1.000000000000000000, 0.9238795325112867385, 1.000000000000000000, 0.9238795325112867385, 1.000000000000000000, 0.9238795325112874046, 0.9999999999999993339 ) ) 
 REPRESENTATION_ITEM ( '' )  );
#1320=CARTESIAN_POINT ( 'NONE',  ( 4.729367062499999719, -31.28125000204839168, 0.000000000000000000 ) ) ;
#1326=CARTESIAN_POINT ( 'NONE',  ( -1.846868145590737420, -24.00000000136559564, 4.458734124999997661 ) ) ;
#1328=CARTESIAN_POINT ( 'NONE',  ( 4.458734124999999437, -23.37500000136559564, -1.846868145590734978 ) ) ;
#1330=CARTESIAN_POINT ( 'NONE',  ( 6.123233995736766282E-16, -20.00000000000000000, -5.000000000000000000 ) ) ;
#1331=ORIENTED_EDGE ( 'NONE', *, *, #15514, .F. ) ;
#1335=CARTESIAN_POINT ( 'NONE',  ( 2.071067811865473285, -30.93750000273118417, -5.000000000000002665 ) ) ;
#1337=CARTESIAN_POINT ( 'NONE',  ( -9.184850993605147944E-16, -22.25000000000000000, 5.000000000000000000 ) ) ;
#1346=CARTESIAN_POINT ( 'NONE',  ( 4.458734124999999437, -26.43750000136559564, 0.000000000000000000 ) ) ;
#1353=CARTESIAN_POINT ( 'NONE',  ( -3.152801135295367096, -26.06250000136559564, -3.152801135295367541 ) ) ;
#1354=DIRECTION ( 'NONE',  ( 0.000000000000000000, 1.000000000000000000, 0.000000000000000000 ) ) ;
#1361=CARTESIAN_POINT ( 'NONE',  ( -2.071067811865478170, -28.31250000000000355, 5.000000000000000000 ) ) ;
#1365=ADVANCED_FACE ( 'NONE', ( #259 ), #12501, .T. ) ;
#1366=CARTESIAN_POINT ( 'NONE',  ( -5.000000000000000888, -28.56250000273118417, 2.071067811865474617 ) ) ;
#1368=CARTESIAN_POINT ( 'NONE',  ( 3.152801135295367541, -30.31250000136559564, -3.152801135295367541 ) ) ;
#1377=CARTESIAN_POINT ( 'NONE',  ( 1.846868145590735200, -31.50000000136559564, -4.458734125000000326 ) ) ;
#1397=CARTESIAN_POINT ( 'NONE',  ( 0.000000000000000000, -32.00000000000000000, 0.000000000000000000 ) ) ;
#1400=CARTESIAN_POINT ( 'NONE',  ( -9.184850993605147944E-16, -30.37500000273118772, 5.000000000000000000 ) ) ;
#1405=CARTESIAN_POINT ( 'NONE',  ( 4.458734124999999437, -25.68750000136559564, 0.000000000000000000 ) ) ;
#1414=ORIENTED_EDGE ( 'NONE', *, *, #10465, .T. ) ;
#1427=CARTESIAN_POINT ( 'NONE',  ( -4.458734125000000326, -27.00000000136559208, -1.846868145590735644 ) ) ;
#1433=ORIENTED_EDGE ( 'NONE', *, *, #292, .F. ) ;
#1434=AXIS2_PLACEMENT_3D ( 'NONE', #9682, #10829, #12021 ) ;
#1435=CARTESIAN_POINT ( 'NONE',  ( 2.730187237215162345E-16, -24.18750000136559564, -4.458734124999999437 ) ) ;
#1439=EDGE_CURVE ( 'NONE', #2989, #10378, #3177, .T. ) ;
#1440=EDGE_CURVE ( 'NONE', #580, #15000, #2895, .T. ) ;
#1442=DIRECTION ( 'NONE',  ( 0.000000000000000000, 0.000000000000000000, 1.000000000000000000 ) ) ;
#1443=PLANE ( 'NONE',  #5897 ) ;
#1445=VECTOR ( 'NONE', #11850, 1000.000000000000000 ) ;
#1446=CARTESIAN_POINT ( 'NONE',  ( -3.535533905932738641, -31.37500000000000000, 3.535533905932737309 ) ) ;
#1447=FACE_OUTER_BOUND ( 'NONE', #829, .T. ) ;
#1449=CARTESIAN_POINT ( 'NONE',  ( -9.184850993605147944E-16, -28.37500000273118772, 5.000000000000000000 ) ) ;
#1451=CARTESIAN_POINT ( 'NONE',  ( 3.152801135295366208, -28.56250000136559564, 3.152801135295367985 ) ) ;
#1453=ORIENTED_EDGE ( 'NONE', *, *, #10965, .T. ) ;
#1455=ORIENTED_EDGE ( 'NONE', *, *, #15652, .F. ) ;
#1459=VECTOR ( 'NONE', #8668, 1000.000000000000114 ) ;
#1460=EDGE_LOOP ( 'NONE', ( #15119, #13685, #4899, #13163 ) ) ;
#1462=LINE ( 'NONE', #6485, #9231 ) ;
#1467=CARTESIAN_POINT ( 'NONE',  ( 1.846868145590736310, -30.87500000136559564, 4.458734124999999437 ) ) ;
#1468=CARTESIAN_POINT ( 'NONE',  ( 4.458734124999999437, -26.50000000136559208, 1.846868145590737864 ) ) ;
#1472=DIRECTION ( 'NONE',  ( -0.000000000000000000, 1.000000000000000000, -0.000000000000000000 ) ) ;
#1480=ORIENTED_EDGE ( 'NONE', *, *, #10379, .T. ) ;
#1483=EDGE_CURVE ( 'NONE', #14678, #10126, #14455, .T. ) ;
#1487=AXIS2_PLACEMENT_3D ( 'NONE', #13513, #11863, #2784 ) ;
#1512=AXIS2_PLACEMENT_3D ( 'NONE', #14485, #8045, #10457 ) ;
#1513=CARTESIAN_POINT ( 'NONE',  ( 3.535533905932736864, -26.12500000000000355, 3.535533905932738641 ) ) ;
#1520=CARTESIAN_POINT ( 'NONE',  ( 3.152801135295367541, -24.31250000136559564, -3.152801135295367541 ) ) ;
#1528=CARTESIAN_POINT ( 'NONE',  ( 4.458734124999999437, -21.50000000136559208, 1.846868145590737864 ) ) ;
#1534=CARTESIAN_POINT ( 'NONE',  ( 5.000000000000000000, -30.00000000000000000, 0.000000000000000000 ) ) ;
#1537=CARTESIAN_POINT ( 'NONE',  ( 3.535533905932738197, -24.00000000273118772, -3.535533905932738197 ) ) ;
#1539=CARTESIAN_POINT ( 'NONE',  ( 3.152801135295367541, -31.31250000136559564, -3.152801135295367541 ) ) ;
#1550=CARTESIAN_POINT ( 'NONE',  ( 2.730187237215162345E-16, -30.43750000136559564, -4.458734124999999437 ) ) ;
#1561=CARTESIAN_POINT ( 'NONE',  ( 4.458734124999999437, -31.43750000136559564, 0.000000000000000000 ) ) ;
#1562=ORIENTED_EDGE ( 'NONE', *, *, #292, .T. ) ;
#1568=CYLINDRICAL_SURFACE ( 'NONE', #10807, 5.000000000000000000 ) ;
#1573=CARTESIAN_POINT ( 'NONE',  ( -35.00000000000000000, 37.00000000000000000, 6.000000000000000000 ) ) ;
#1576=DIRECTION ( 'NONE',  ( 0.000000000000000000, -0.000000000000000000, 1.000000000000000000 ) ) ;
#1579=ORIENTED_EDGE ( 'NONE', *, *, #8085, .F. ) ;
#1583=( BOUNDED_CURVE ( )  B_SPLINE_CURVE ( 2, ( #3767, #3854, #1513, #12646, #4002, #12480, #10084, #15011, #14935 ),
 .UNSPECIFIED., .F., .F. ) 
 B_SPLINE_CURVE_WITH_KNOTS ( ( 3, 2, 2, 2, 3 ),
 ( 0.5749999999999998446, 0.5874999999999999112, 0.5999999999999998668, 0.6124999999999999334, 0.6249999999999998890 ),
 .UNSPECIFIED. ) 
 CURVE ( )  GEOMETRIC_REPRESENTATION_ITEM ( )  RATIONAL_B_SPLINE_CURVE ( ( 1.000000000000000666, 0.9238795325112860723, 1.000000000000000000, 0.9238795325112867385, 1.000000000000000000, 0.9238795325112867385, 1.000000000000000000, 0.9238795325112874046, 0.9999999999999993339 ) ) 
 REPRESENTATION_ITEM ( '' )  );
#1591=CARTESIAN_POINT ( 'NONE',  ( 2.071067811865482611, -28.81250000000000000, -4.999999999999992895 ) ) ;
#1592=CARTESIAN_POINT ( 'NONE',  ( -4.458734125000000326, -24.00000000136559564, -1.846868145590735644 ) ) ;
#1593=EDGE_CURVE ( 'NONE', #2810, #7938, #11124, .T. ) ;
#1599=CARTESIAN_POINT ( 'NONE',  ( 4.458734125000000326, -22.37500000136559564, -1.846868145590734978 ) ) ;
#1602=CARTESIAN_POINT ( 'NONE',  ( -3.535533905932738641, -28.37500000000000000, 3.535533905932737309 ) ) ;
#1603=LINE ( 'NONE', #168, #7207 ) ;
#1604=DIRECTION ( 'NONE',  ( 0.000000000000000000, 0.000000000000000000, -1.000000000000000000 ) ) ;
#1606=CARTESIAN_POINT ( 'NONE',  ( 5.000000000000000000, -28.06250000000000000, 2.071067811865478614 ) ) ;
#1609=CARTESIAN_POINT ( 'NONE',  ( 3.535533905932736864, -25.25000000273118417, 3.535533905932738641 ) ) ;
#1612=CARTESIAN_POINT ( 'NONE',  ( 3.152801135295366208, -27.56250000136559564, 3.152801135295367985 ) ) ;
#1625=CARTESIAN_POINT ( 'NONE',  ( 4.458734124999999437, -30.68750000136559564, 0.000000000000000000 ) ) ;
#1645=DIRECTION ( 'NONE',  ( 0.000000000000000000, 0.000000000000000000, -1.000000000000000000 ) ) ;
#1646=CARTESIAN_POINT ( 'NONE',  ( -8.190561711645485556E-16, -21.93750000136559208, 4.458734124999999437 ) ) ;
#1655=DIRECTION ( 'NONE',  ( -0.000000000000000000, 1.000000000000000000, -0.000000000000000000 ) ) ;
#1657=FACE_OUTER_BOUND ( 'NONE', #13410, .T. ) ;
#1663=DIRECTION ( 'NONE',  ( 0.000000000000000000, -0.000000000000000000, 1.000000000000000000 ) ) ;
#1667=CARTESIAN_POINT ( 'NONE',  ( 0.000000000000000000, -20.00000000000000000, 0.000000000000000000 ) ) ;
#1674=( BOUNDED_SURFACE ( )  B_SPLINE_SURFACE ( 1, 2, ( 
 ( #1561, #10216, #8769, #204, #6572, #5365, #11411, #2845, #436, #7800, #10304, #2095, #8269, #13306, #4601, #8338, #2249, #2020, #3009, #7040, #12771, #9681, #11574, #14540, #895, #11941, #7119, #5898, #7958, #9164, #10827, #5815, #12020, #3319, #3389, #15769, #13161, #7203, #1042, #10750, #2169, #12860, #8415, #10377, #970, #2923, #5735, #4524, #4680, #15687, #4221, #15841, #13230, #10673, #815, #1716, #14082, #528, #9539, #6968, #7873, #15605, #6664, #3459, #9604, #12104, #14467, #10900, #15305, #5444, #5977, #11869, #9458, #4759, #14390, #3700, #8730, #6140, #13392, #13458, #11138, #6301, #13635, #11067, #77, #6381, #1353, #11216, #163, #12419, #2645, #3784, #6055, #2399, #7350, #12175, #14862, #14704, #2563, #1277, #7516, #12257, #4843, #5080, #3626, #1115, #10014, #4, #3868, #11300, #3539, #4995, #8807, #9922, #7596, #12494, #1435, #7274, #14952, #8570, #13711, #252, #5168, #1196, #14619, #8496, #2330, #10982, #15922, #9769, #4920, #12342, #9846, #14777, #6224, #8646, #13543, #2477, #7437, #7768, #4018, #6778, #6537, #10342, #12659, #1599, #8887, #328, #2725, #11533, #15099, #639, #11452, #15024, #10412, #15269, #11611, #485, #1833, #1528, #10097 ),
 ( #15188, #4183, #399, #13789, #8968, #6619, #1762, #9129, #5324, #5407, #11687, #12816, #6709, #562, #7916, #14129, #14040, #6465, #13879, #2812, #7680, #2966, #10174, #5483, #12734, #15348, #10263, #5237, #4266, #4104, #12579, #9208, #9053, #3058, #3939, #11377, #8004, #12901, #13956, #2889, #7840, #1676, #14215, #2076, #15512, #2150, #13209, #8320, #9362, #14520, #9588, #15751, #7099, #4581, #8393, #719, #3295, #7021, #5645, #8247, #10586, #11767, #11923, #11849, #3209, #4429, #2227, #1997, #10729, #4664, #14287, #8158, #9439, #15432, #12082, #3135, #950, #13143, #4502, #9519, #12000, #13059, #6947, #5877, #14366, #14451, #5716, #5792, #10811, #10654, #3440, #13286, #15586, #3373, #796, #7181, #12977, #5564, #10500, #875, #15667, #4352, #9290, #6860, #8081, #1913, #1173, #139, #4903, #6037, #6115, #6119, #11194, #2458, #2382, #14841, #11045, #8473, #7258, #14685, #13612, #3606, #12158, #12235, #5059, #14929, #7415, #9995, #13374, #11121, #9828, #3849, #3519, #1026, #1096, #10957, #60, #4975, #2544, #12400, #14758, #8553, #3763, #13522, #3681, #2313, #10881, #15901, #12319, #8790, #13693, #4820, #4740, #9747, #13442, #2627, #1258, #14596, #7578, #8709, #8628 ) ),
 .UNSPECIFIED., .F., .F., .F. ) 
 B_SPLINE_SURFACE_WITH_KNOTS ( ( 2, 2 ),
 ( 3, 2, 2, 2, 2, 2, 2, 2, 2, 2, 2, 2, 2, 2, 2, 2, 2, 2, 2, 2, 2, 2, 2, 2, 2, 2, 2, 2, 2, 2, 2, 2, 2, 2, 2, 2, 2, 2, 2, 2, 2, 2, 2, 2, 2, 2, 2, 2, 2, 2, 2, 2, 2, 2, 2, 2, 2, 2, 2, 2, 2, 2, 2, 2, 2, 2, 2, 2, 2, 2, 2, 2, 2, 2, 2, 2, 2, 2, 2, 2, 3 ),
 ( 0.000000000000000000, 1.000000000000000000 ),
 ( 0.000000000000000000, 0.01250000000000000069, 0.02500000000000000139, 0.03749999999999999861, 0.05000000000000000278, 0.06250000000000000000, 0.07499999999999999722, 0.08749999999999999445, 0.1000000000000000056, 0.1125000000000000028, 0.1250000000000000000, 0.1375000000000000111, 0.1499999999999999944, 0.1625000000000000056, 0.1749999999999999889, 0.1875000000000000000, 0.2000000000000000111, 0.2124999999999999944, 0.2250000000000000056, 0.2374999999999999889, 0.2500000000000000000, 0.2625000000000000111, 0.2750000000000000222, 0.2874999999999999778, 0.2999999999999999889, 0.3125000000000000000, 0.3250000000000000111, 0.3375000000000000222, 0.3499999999999999778, 0.3624999999999999889, 0.3750000000000000000, 0.3875000000000000111, 0.4000000000000000222, 0.4124999999999999778, 0.4249999999999999889, 0.4375000000000000000, 0.4500000000000000111, 0.4625000000000000222, 0.4749999999999999778, 0.4874999999999999889, 0.5000000000000000000, 0.5124999999999999556, 0.5250000000000000222, 0.5374999999999999778, 0.5500000000000000444, 0.5625000000000000000, 0.5749999999999999556, 0.5875000000000000222, 0.5999999999999999778, 0.6125000000000000444, 0.6250000000000000000, 0.6374999999999999556, 0.6500000000000000222, 0.6624999999999999778, 0.6750000000000000444, 0.6875000000000000000, 0.6999999999999999556, 0.7125000000000000222, 0.7249999999999999778, 0.7375000000000000444, 0.7500000000000000000, 0.7624999999999999556, 0.7750000000000000222, 0.7874999999999999778, 0.8000000000000000444, 0.8125000000000000000, 0.8249999999999999556, 0.8375000000000000222, 0.8499999999999999778, 0.8625000000000000444, 0.8750000000000000000, 0.8874999999999999556, 0.9000000000000000222, 0.9124999999999999778, 0.9250000000000000444, 0.9375000000000000000, 0.9499999999999999556, 0.9625000000000000222, 0.9749999999999999778, 0.9875000000000000444, 1.000000000000000000 ),
 .UNSPECIFIED. ) 
 GEOMETRIC_REPRESENTATION_ITEM ( )  RATIONAL_B_SPLINE_SURFACE ( (
 ( 1.000000000000000000, 0.9238795325112867385, 1.000000000000000000, 0.9238795325112867385, 1.000000000000000000, 0.9238795325112867385, 1.000000000000000000, 0.9238795325112867385, 1.000000000000000000, 0.9238795325112867385, 1.000000000000000000, 0.9238795325112867385, 1.000000000000000000, 0.9238795325112867385, 1.000000000000000000, 0.9238795325112867385, 1.000000000000000000, 0.9238795325112867385, 1.000000000000000000, 0.9238795325112867385, 1.000000000000000000, 0.9238795325112867385, 1.000000000000000000, 0.9238795325112867385, 1.000000000000000000, 0.9238795325112867385, 1.000000000000000000, 0.9238795325112867385, 1.000000000000000000, 0.9238795325112867385, 1.000000000000000000, 0.9238795325112867385, 1.000000000000000000, 0.9238795325112867385, 1.000000000000000000, 0.9238795325112867385, 1.000000000000000000, 0.9238795325112867385, 1.000000000000000000, 0.9238795325112867385, 1.000000000000000000, 0.9238795325112867385, 1.000000000000000000, 0.9238795325112867385, 1.000000000000000000, 0.9238795325112867385, 1.000000000000000000, 0.9238795325112867385, 1.000000000000000000, 0.9238795325112867385, 1.000000000000000000, 0.9238795325112867385, 1.000000000000000000, 0.9238795325112867385, 1.000000000000000000, 0.9238795325112867385, 1.000000000000000000, 0.9238795325112867385, 1.000000000000000000, 0.9238795325112867385, 1.000000000000000000, 0.9238795325112867385, 1.000000000000000000, 0.9238795325112867385, 1.000000000000000000, 0.9238795325112867385, 1.000000000000000000, 0.9238795325112867385, 1.000000000000000000, 0.9238795325112867385, 1.000000000000000000, 0.9238795325112867385, 1.000000000000000000, 0.9238795325112867385, 1.000000000000000000, 0.9238795325112867385, 1.000000000000000000, 0.9238795325112867385, 1.000000000000000000, 0.9238795325112867385, 1.000000000000000000, 0.9238795325112867385, 1.000000000000000000, 0.9238795325112867385, 1.000000000000000000, 0.9238795325112867385, 1.000000000000000000, 0.9238795325112867385, 1.000000000000000000, 0.9238795325112867385, 1.000000000000000000, 0.9238795325112867385, 1.000000000000000000, 0.9238795325112867385, 1.000000000000000000, 0.9238795325112867385, 1.000000000000000000, 0.9238795325112867385, 1.000000000000000000, 0.9238795325112867385, 1.000000000000000000, 0.9238795325112867385, 1.000000000000000000, 0.9238795325112867385, 1.000000000000000000, 0.9238795325112867385, 1.000000000000000000, 0.9238795325112867385, 1.000000000000000000, 0.9238795325112867385, 1.000000000000000000, 0.9238795325112867385, 1.000000000000000000, 0.9238795325112867385, 1.000000000000000000, 0.9238795325112867385, 1.000000000000000000, 0.9238795325112867385, 1.000000000000000000, 0.9238795325112867385, 1.000000000000000000, 0.9238795325112867385, 1.000000000000000000, 0.9238795325112867385, 1.000000000000000000, 0.9238795325112867385, 1.000000000000000000, 0.9238795325112867385, 1.000000000000000000, 0.9238795325112867385, 1.000000000000000000, 0.9238795325112867385, 1.000000000000000000, 0.9238795325112867385, 1.000000000000000000, 0.9238795325112867385, 1.000000000000000000, 0.9238795325112867385, 1.000000000000000000, 0.9238795325112867385, 1.000000000000000000, 0.9238795325112867385, 1.000000000000000000, 0.9238795325112867385, 1.000000000000000000, 0.9238795325112867385, 1.000000000000000000, 0.9238795325112867385, 1.000000000000000000, 0.9238795325112867385, 1.000000000000000000, 0.9238795325112867385, 1.000000000000000000, 0.9238795325112867385, 1.000000000000000000, 0.9238795325112867385, 1.000000000000000000, 0.9238795325112867385, 1.000000000000000000, 0.9238795325112867385, 1.000000000000000000),
 ( 1.000000000000000000, 0.9238795325112867385, 1.000000000000000000, 0.9238795325112867385, 1.000000000000000000, 0.9238795325112867385, 1.000000000000000000, 0.9238795325112867385, 1.000000000000000000, 0.9238795325112867385, 1.000000000000000000, 0.9238795325112867385, 1.000000000000000000, 0.9238795325112867385, 1.000000000000000000, 0.9238795325112867385, 1.000000000000000000, 0.9238795325112867385, 1.000000000000000000, 0.9238795325112867385, 1.000000000000000000, 0.9238795325112867385, 1.000000000000000000, 0.9238795325112867385, 1.000000000000000000, 0.9238795325112867385, 1.000000000000000000, 0.9238795325112867385, 1.000000000000000000, 0.9238795325112867385, 1.000000000000000000, 0.9238795325112867385, 1.000000000000000000, 0.9238795325112867385, 1.000000000000000000, 0.9238795325112867385, 1.000000000000000000, 0.9238795325112867385, 1.000000000000000000, 0.9238795325112867385, 1.000000000000000000, 0.9238795325112867385, 1.000000000000000000, 0.9238795325112867385, 1.000000000000000000, 0.9238795325112867385, 1.000000000000000000, 0.9238795325112867385, 1.000000000000000000, 0.9238795325112867385, 1.000000000000000000, 0.9238795325112867385, 1.000000000000000000, 0.9238795325112867385, 1.000000000000000000, 0.9238795325112867385, 1.000000000000000000, 0.9238795325112867385, 1.000000000000000000, 0.9238795325112867385, 1.000000000000000000, 0.9238795325112867385, 1.000000000000000000, 0.9238795325112867385, 1.000000000000000000, 0.9238795325112867385, 1.000000000000000000, 0.9238795325112867385, 1.000000000000000000, 0.9238795325112867385, 1.000000000000000000, 0.9238795325112867385, 1.000000000000000000, 0.9238795325112867385, 1.000000000000000000, 0.9238795325112867385, 1.000000000000000000, 0.9238795325112867385, 1.000000000000000000, 0.9238795325112867385, 1.000000000000000000, 0.9238795325112867385, 1.000000000000000000, 0.9238795325112867385, 1.000000000000000000, 0.9238795325112867385, 1.000000000000000000, 0.9238795325112867385, 1.000000000000000000, 0.9238795325112867385, 1.000000000000000000, 0.9238795325112867385, 1.000000000000000000, 0.9238795325112867385, 1.000000000000000000, 0.9238795325112867385, 1.000000000000000000, 0.9238795325112867385, 1.000000000000000000, 0.9238795325112867385, 1.000000000000000000, 0.9238795325112867385, 1.000000000000000000, 0.9238795325112867385, 1.000000000000000000, 0.9238795325112867385, 1.000000000000000000, 0.9238795325112867385, 1.000000000000000000, 0.9238795325112867385, 1.000000000000000000, 0.9238795325112867385, 1.000000000000000000, 0.9238795325112867385, 1.000000000000000000, 0.9238795325112867385, 1.000000000000000000, 0.9238795325112867385, 1.000000000000000000, 0.9238795325112867385, 1.000000000000000000, 0.9238795325112867385, 1.000000000000000000, 0.9238795325112867385, 1.000000000000000000, 0.9238795325112867385, 1.000000000000000000, 0.9238795325112867385, 1.000000000000000000, 0.9238795325112867385, 1.000000000000000000, 0.9238795325112867385, 1.000000000000000000, 0.9238795325112867385, 1.000000000000000000, 0.9238795325112867385, 1.000000000000000000, 0.9238795325112867385, 1.000000000000000000, 0.9238795325112867385, 1.000000000000000000, 0.9238795325112867385, 1.000000000000000000, 0.9238795325112867385, 1.000000000000000000, 0.9238795325112867385, 1.000000000000000000, 0.9238795325112867385, 1.000000000000000000, 0.9238795325112867385, 1.000000000000000000, 0.9238795325112867385, 1.000000000000000000, 0.9238795325112867385, 1.000000000000000000, 0.9238795325112867385, 1.000000000000000000, 0.9238795325112867385, 1.000000000000000000, 0.9238795325112867385, 1.000000000000000000) ) ) 
 REPRESENTATION_ITEM ( '' )  SURFACE ( )  );
#1676=CARTESIAN_POINT ( 'NONE',  ( -4.458734125000001214, -29.12500000136559919, 1.846868145590734089 ) ) ;
#1678=AXIS2_PLACEMENT_3D ( 'NONE', #4647, #9572, #6017 ) ;
#1683=EDGE_CURVE ( 'NONE', #13499, #13973, #4204, .T. ) ;
#1688=CARTESIAN_POINT ( 'NONE',  ( 2.071067811865476394, -29.18750000000000711, 5.000000000000000000 ) ) ;
#1689=AXIS2_PLACEMENT_3D ( 'NONE', #3622, #7512, #12252 ) ;
#1691=CARTESIAN_POINT ( 'NONE',  ( -2.071067811865447084, -21.81250000273119483, -5.000000000000029310 ) ) ;
#1693=CARTESIAN_POINT ( 'NONE',  ( -3.535533905932737309, -25.75000000273118417, -3.535533905932738197 ) ) ;
#1695=CARTESIAN_POINT ( 'NONE',  ( -8.190561711645485556E-16, -27.68750000136559564, 4.458734124999999437 ) ) ;
#1704=VECTOR ( 'NONE', #6466, 1000.000000000000000 ) ;
#1716=CARTESIAN_POINT ( 'NONE',  ( -4.458734125000000326, -28.00000000136559564, -1.846868145590735644 ) ) ;
#1738=CARTESIAN_POINT ( 'NONE',  ( 3.061616997868383141E-16, -24.75000000000000000, -5.000000000000000000 ) ) ;
#1744=CARTESIAN_POINT ( 'NONE',  ( 7.347880794884120722E-16, -13.00000000000000178, 6.000000000000000888 ) ) ;
#1751=CARTESIAN_POINT ( 'NONE',  ( 3.152801135295367541, -22.31250000136559564, -3.152801135295367541 ) ) ;
#1760=VECTOR ( 'NONE', #11899, 1000.000000000000000 ) ;
#1762=CARTESIAN_POINT ( 'NONE',  ( -3.152801135295367096, -31.31250000136559564, -3.152801135295367541 ) ) ;
#1770=CARTESIAN_POINT ( 'NONE',  ( 3.535533905932736864, -26.12500000000000355, 3.535533905932738641 ) ) ;
#1772=CARTESIAN_POINT ( 'NONE',  ( 35.00000000000000000, 37.00000000000000000, -5.999999999999991118 ) ) ;
#1774=CARTESIAN_POINT ( 'NONE',  ( 3.535533905932738197, -25.00000000273118417, -3.535533905932738197 ) ) ;
#1777=CARTESIAN_POINT ( 'NONE',  ( -1.846868145590737420, -24.75000000136559564, 4.458734124999997661 ) ) ;
#1786=VECTOR ( 'NONE', #14776, 1000.000000000000000 ) ;
#1788=CARTESIAN_POINT ( 'NONE',  ( 0.000000000000000000, -20.00000000000000000, 0.000000000000000000 ) ) ;
#1789=FACE_OUTER_BOUND ( 'NONE', #851, .T. ) ;
#1790=CARTESIAN_POINT ( 'NONE',  ( -1.846868145590734756, -26.37500000136559564, -4.458734125000000326 ) ) ;
#1797=SHAPE_REPRESENTATION_RELATIONSHIP ( 'NONE' , 'NONE' ,  #7495, #10261 ) ;
#1802=DIRECTION ( 'NONE',  ( -0.000000000000000000, -1.000000000000000000, -0.000000000000000000 ) ) ;
#1817=DIRECTION ( 'NONE',  ( 0.000000000000000000, 0.000000000000000000, 1.000000000000000000 ) ) ;
#1820=EDGE_CURVE ( 'NONE', #8371, #10126, #2129, .T. ) ;
#1821=CARTESIAN_POINT ( 'NONE',  ( 3.535533905932736864, -26.25000000273118417, 3.535533905932738641 ) ) ;
#1825=CARTESIAN_POINT ( 'NONE',  ( 6.123233995736766282E-16, -20.00000000000000000, -5.000000000000000000 ) ) ;
#1827=CARTESIAN_POINT ( 'NONE',  ( 3.152801135295366208, -23.56250000136559564, 3.152801135295367985 ) ) ;
#1833=CARTESIAN_POINT ( 'NONE',  ( 3.152801135295366208, -21.56250000136559208, 3.152801135295367985 ) ) ;
#1835=ORIENTED_EDGE ( 'NONE', *, *, #1935, .T. ) ;
#1843=CARTESIAN_POINT ( 'NONE',  ( -2.071067811865475061, -24.68750000000000355, -5.000000000000000888 ) ) ;
#1847=CARTESIAN_POINT ( 'NONE',  ( -2.071067811865475061, -23.81250000273118772, -5.000000000000000888 ) ) ;
#1849=CARTESIAN_POINT ( 'NONE',  ( 4.458734124999997661, -25.50000000136559919, 1.846868145590737864 ) ) ;
#1853=CARTESIAN_POINT ( 'NONE',  ( -35.00000000000000000, 37.00000000000000000, 2.649999999999985700 ) ) ;
#1860=CARTESIAN_POINT ( 'NONE',  ( 1.846868145590736310, -25.87500000136559919, 4.458734124999999437 ) ) ;
#1867=ORIENTED_EDGE ( 'NONE', *, *, #12222, .T. ) ;
#1904=CARTESIAN_POINT ( 'NONE',  ( 4.458734124999999437, -28.68750000136559564, 0.000000000000000000 ) ) ;
#1913=CARTESIAN_POINT ( 'NONE',  ( -4.458734125000001214, -25.12500000136559564, 1.846868145590734089 ) ) ;
#1914=LINE ( 'NONE', #2077, #1445 ) ;
#1920=CARTESIAN_POINT ( 'NONE',  ( 3.061616997868383141E-16, -25.75000000000000355, -5.000000000000000000 ) ) ;
#1924=CARTESIAN_POINT ( 'NONE',  ( 3.152801135295367541, -29.31250000136559208, -3.152801135295367541 ) ) ;
#1927=CARTESIAN_POINT ( 'NONE',  ( 4.458734124999999437, -27.43750000136559564, 0.000000000000000000 ) ) ;
#1935=EDGE_CURVE ( 'NONE', #15134, #2381, #9873, .T. ) ;
#1937=CARTESIAN_POINT ( 'NONE',  ( -5.000000000000000888, -24.68750000273118772, -2.071067811865475949 ) ) ;
#1940=CARTESIAN_POINT ( 'NONE',  ( -24.26932219902320043, 20.00000000000000000, 5.999999999999998224 ) ) ;
#1942=CARTESIAN_POINT ( 'NONE',  ( 4.458734125000000326, -25.62500000136559564, -1.846868145590734978 ) ) ;
#1948=ORIENTED_EDGE ( 'NONE', *, *, #5298, .T. ) ;
#1951=EDGE_LOOP ( 'NONE', ( #3605, #5125, #8000, #7015, #1453, #6014, #15457, #9265, #5583, #6594, #755, #6379 ) ) ;
#1953=EDGE_CURVE ( 'NONE', #13669, #12414, #6650, .T. ) ;
#1958=CARTESIAN_POINT ( 'NONE',  ( 35.00000000000000000, 40.00000000000000000, 2.649999999999983924 ) ) ;
#1965=CARTESIAN_POINT ( 'NONE',  ( 4.729367062499999719, -21.84375000068279604, 0.000000000000000000 ) ) ;
#1968=CARTESIAN_POINT ( 'NONE',  ( 6.000000000000000000, -13.00000000000000178, -1.500000000000000000 ) ) ;
#1973=CARTESIAN_POINT ( 'NONE',  ( -9.184850993605147944E-16, -27.25000000000000000, 5.000000000000000000 ) ) ;
#1978=CYLINDRICAL_SURFACE ( 'NONE', #13067, 5.000000000000000000 ) ;
#1981=FACE_OUTER_BOUND ( 'NONE', #7072, .T. ) ;
#1984=CARTESIAN_POINT ( 'NONE',  ( 5.000000000000000888, -22.93749999999999645, -2.071067811865475505 ) ) ;
#1988=CARTESIAN_POINT ( 'NONE',  ( -8.190561711645485556E-16, -27.93750000136559564, 4.458734124999999437 ) ) ;
#1993=ORIENTED_EDGE ( 'NONE', *, *, #6721, .F. ) ;
#1997=CARTESIAN_POINT ( 'NONE',  ( 1.846868145590735200, -27.50000000136559208, -4.458734125000000326 ) ) ;
#2000=DIRECTION ( 'NONE',  ( -0.000000000000000000, 1.000000000000000000, -0.000000000000000000 ) ) ;
#2006=CARTESIAN_POINT ( 'NONE',  ( 5.000000000000000000, -24.06250000000000000, 2.071067811865478614 ) ) ;
#2011=CARTESIAN_POINT ( 'NONE',  ( -5.000000000000000888, -21.56250000273118772, 2.071067811865474617 ) ) ;
#2012=ORIENTED_EDGE ( 'NONE', *, *, #4980, .F. ) ;
#2013=CARTESIAN_POINT ( 'NONE',  ( 4.458734124999997661, -23.50000000136559564, 1.846868145590737864 ) ) ;
#2015=ORIENTED_EDGE ( 'NONE', *, *, #11671, .T. ) ;
#2020=CARTESIAN_POINT ( 'NONE',  ( 4.458734125000000326, -30.37500000136559564, -1.846868145590734978 ) ) ;
#2022=ORIENTED_EDGE ( 'NONE', *, *, #3556, .F. ) ;
#2026=CARTESIAN_POINT ( 'NONE',  ( 3.061616997868383141E-16, -23.75000000000000000, -5.000000000000000000 ) ) ;
#2027=CARTESIAN_POINT ( 'NONE',  ( 3.152801135295366208, -26.81250000136559564, 3.152801135295367985 ) ) ;
#2029=CARTESIAN_POINT ( 'NONE',  ( 0.000000000000000000, 20.00000000000000000, 0.000000000000000000 ) ) ;
#2031=CARTESIAN_POINT ( 'NONE',  ( 5.000000000000000000, -31.00000000000000000, 0.000000000000000000 ) ) ;
#2036=VERTEX_POINT ( 'NONE', #3668 ) ;
#2037=DIRECTION ( 'NONE',  ( 0.000000000000000000, -1.000000000000000000, 0.000000000000000000 ) ) ;
#2056=VERTEX_POINT ( 'NONE', #6022 ) ;
#2065=CARTESIAN_POINT ( 'NONE',  ( -5.000000000000000888, -29.56250000273118417, 2.071067811865474617 ) ) ;
#2069=CARTESIAN_POINT ( 'NONE',  ( -1.846868145590734756, -29.37500000136559564, -4.458734124999999437 ) ) ;
#2074=VERTEX_POINT ( 'NONE', #5863 ) ;
#2076=CARTESIAN_POINT ( 'NONE',  ( -1.846868145590737420, -29.00000000136559564, 4.458734124999999437 ) ) ;
#2077=CARTESIAN_POINT ( 'NONE',  ( 0.000000000000000000, -20.00000000000000000, 5.000000000000000000 ) ) ;
#2086=CARTESIAN_POINT ( 'NONE',  ( -5.000000000000000888, -21.56250000273118772, 2.071067811865474617 ) ) ;
#2088=CARTESIAN_POINT ( 'NONE',  ( -1.846868145590737420, -30.75000000136559564, 4.458734124999999437 ) ) ;
#2090=CARTESIAN_POINT ( 'NONE',  ( -3.152801135295367985, -23.81250000136559564, 3.152801135295367096 ) ) ;
#2095=CARTESIAN_POINT ( 'NONE',  ( -1.846868145590737420, -30.75000000136559564, 4.458734124999999437 ) ) ;
#2103=CARTESIAN_POINT ( 'NONE',  ( 4.458734124999999437, -26.75000000136559564, 1.846868145590737864 ) ) ;
#2106=CARTESIAN_POINT ( 'NONE',  ( 3.535533905932738197, -31.00000000273118772, -3.535533905932738197 ) ) ;
#2112=EDGE_CURVE ( 'NONE', #14535, #8138, #5437, .T. ) ;
#2118=CARTESIAN_POINT ( 'NONE',  ( 2.071067811865503927, -21.93750000273119127, -4.999999999999971578 ) ) ;
#2120=CARTESIAN_POINT ( 'NONE',  ( -5.000000000000000888, -22.56250000000000000, -2.071067811865475949 ) ) ;
#2123=VERTEX_POINT ( 'NONE', #8918 ) ;
#2124=AXIS2_PLACEMENT_3D ( 'NONE', #11950, #9545, #14472 ) ;
#2126=CARTESIAN_POINT ( 'NONE',  ( 3.535533905932736864, -23.25000000273118772, 3.535533905932738641 ) ) ;
#2129=CIRCLE ( 'NONE', #11669, 2.649999999999985700 ) ;
#2136=CARTESIAN_POINT ( 'NONE',  ( 35.00000000000000000, 37.00000000000000000, -8.572527594031472993E-15 ) ) ;
#2139=CARTESIAN_POINT ( 'NONE',  ( 7.347880794884120722E-16, -11.00000000000000178, 6.000000000000000888 ) ) ;
#2141=CARTESIAN_POINT ( 'NONE',  ( -8.190561711645485556E-16, -29.93750000136559564, 4.458734124999999437 ) ) ;
#2143=VERTEX_POINT ( 'NONE', #10368 ) ;
#2144=DIRECTION ( 'NONE',  ( 0.000000000000000000, 0.000000000000000000, -1.000000000000000000 ) ) ;
#2149=VECTOR ( 'NONE', #15502, 1000.000000000000000 ) ;
#2150=CARTESIAN_POINT ( 'NONE',  ( 1.846868145590736310, -28.87500000136559564, 4.458734124999999437 ) ) ;
#2154=CARTESIAN_POINT ( 'NONE',  ( -35.00000000000000000, 40.00000000000000000, -2.649999999999992806 ) ) ;
#2161=CARTESIAN_POINT ( 'NONE',  ( 3.535533905932736864, -22.25000000273118417, 3.535533905932738641 ) ) ;
#2169=CARTESIAN_POINT ( 'NONE',  ( -4.458734124999999437, -28.93750000136559564, -5.460374474430324690E-16 ) ) ;
#2177=CARTESIAN_POINT ( 'NONE',  ( -3.152801135295367096, -24.31250000136559564, -3.152801135295367541 ) ) ;
#2190=VERTEX_POINT ( 'NONE', #14165 ) ;
#2214=CARTESIAN_POINT ( 'NONE',  ( -9.184850993605147944E-16, -29.37500000273118417, 5.000000000000000000 ) ) ;
#2216=CARTESIAN_POINT ( 'NONE',  ( -9.184850993605147944E-16, -24.25000000000000000, 5.000000000000000000 ) ) ;
#2218=CARTESIAN_POINT ( 'NONE',  ( 4.458734124999999437, -29.62500000136559208, -1.846868145590734978 ) ) ;
#2227=CARTESIAN_POINT ( 'NONE',  ( 3.152801135295367541, -27.56250000136559564, -3.152801135295367541 ) ) ;
#2240=ADVANCED_FACE ( 'NONE', ( #12115 ), #4615, .T. ) ;
#2241=CARTESIAN_POINT ( 'NONE',  ( 4.458734124999999437, -29.43750000136559208, 0.000000000000000000 ) ) ;
#2249=CARTESIAN_POINT ( 'NONE',  ( 4.458734124999999437, -30.43750000136559564, 0.000000000000000000 ) ) ;
#2259=CARTESIAN_POINT ( 'NONE',  ( 4.458734124999999437, -22.68750000136559564, 0.000000000000000000 ) ) ;
#2261=EDGE_CURVE ( 'NONE', #2143, #2783, #3919, .T. ) ;
#2265=DIRECTION ( 'NONE',  ( 1.000000000000000000, 0.000000000000000000, 0.000000000000000000 ) ) ;
#2271=FACE_OUTER_BOUND ( 'NONE', #5958, .T. ) ;
#2275=CARTESIAN_POINT ( 'NONE',  ( -3.535533905932738641, -26.37500000000000355, 3.535533905932737309 ) ) ;
#2284=DIRECTION ( 'NONE',  ( -0.000000000000000000, 1.000000000000000000, -0.000000000000000000 ) ) ;
#2285=CARTESIAN_POINT ( 'NONE',  ( 3.061616997868383141E-16, -21.87500000273118772, -4.999999999999999112 ) ) ;
#2292=VERTEX_POINT ( 'NONE', #7214 ) ;
#2302=CARTESIAN_POINT ( 'NONE',  ( -2.071067811865489272, -29.81250000273117706, -4.999999999999985789 ) ) ;
#2304=CARTESIAN_POINT ( 'NONE',  ( -5.000000000000000888, -24.56250000000000000, -2.071067811865475949 ) ) ;
#2305=CARTESIAN_POINT ( 'NONE',  ( -3.535533905932737309, -22.75000000273118772, -3.535533905932738197 ) ) ;
#2306=CARTESIAN_POINT ( 'NONE',  ( 4.458734124999997661, -25.75000000136559564, 1.846868145590737864 ) ) ;
#2313=CARTESIAN_POINT ( 'NONE',  ( 4.458734125000000326, -22.62500000136559564, -1.846868145590734978 ) ) ;
#2319=CARTESIAN_POINT ( 'NONE',  ( -9.184850993605147944E-16, -22.25000000000000000, 5.000000000000000000 ) ) ;
#2322=CARTESIAN_POINT ( 'NONE',  ( -2.071067811865463959, -27.31250000000000000, 5.000000000000013323 ) ) ;
#2323=CARTESIAN_POINT ( 'NONE',  ( -4.458734125000001214, -24.87500000136559919, 1.846868145590734089 ) ) ;
#2325=EDGE_LOOP ( 'NONE', ( #4394, #13278, #3117, #12707, #15185, #9385, #5150, #12361, #3224, #6361 ) ) ;
#2326=CARTESIAN_POINT ( 'NONE',  ( -9.184850993605147944E-16, -29.25000000000000000, 5.000000000000000000 ) ) ;
#2329=DIRECTION ( 'NONE',  ( 1.000000000000000000, 0.000000000000000000, -1.239088197126290570E-16 ) ) ;
#2330=CARTESIAN_POINT ( 'NONE',  ( 3.152801135295366208, -23.56250000136559564, 3.152801135295367985 ) ) ;
#2331=CARTESIAN_POINT ( 'NONE',  ( -9.184850993605147944E-16, -23.25000000000000000, 5.000000000000000000 ) ) ;
#2333=FACE_BOUND ( 'NONE', #10709, .T. ) ;
#2339=CARTESIAN_POINT ( 'NONE',  ( 1.846868145590736310, -24.87500000136559919, 4.458734124999999437 ) ) ;
#2342=CARTESIAN_POINT ( 'NONE',  ( 3.535533905932736864, -31.12500000000000000, 3.535533905932738641 ) ) ;
#2346=ORIENTED_EDGE ( 'NONE', *, *, #6446, .T. ) ;
#2349=ORIENTED_EDGE ( 'NONE', *, *, #12452, .T. ) ;
#2353=CARTESIAN_POINT ( 'NONE',  ( 5.000000000000000000, -28.00000000000000000, 0.000000000000000000 ) ) ;
#2356=DIRECTION ( 'NONE',  ( 0.000000000000000000, -0.000000000000000000, -1.000000000000000000 ) ) ;
#2364=EDGE_CURVE ( 'NONE', #5212, #2989, #11952, .T. ) ;
#2374=CARTESIAN_POINT ( 'NONE',  ( 3.152801135295366208, -26.81250000136559564, 3.152801135295367985 ) ) ;
#2381=VERTEX_POINT ( 'NONE', #13721 ) ;
#2382=CARTESIAN_POINT ( 'NONE',  ( 3.152801135295367541, -24.56250000136559564, -3.152801135295367541 ) ) ;
#2388=CARTESIAN_POINT ( 'NONE',  ( 2.071067811865476394, -22.18749999999999645, 5.000000000000000000 ) ) ;
#2390=LINE ( 'NONE', #2481, #3182 ) ;
#2392=CARTESIAN_POINT ( 'NONE',  ( -8.190561711645485556E-16, -25.68750000136559564, 4.458734124999999437 ) ) ;
#2395=CARTESIAN_POINT ( 'NONE',  ( 3.061616997868383141E-16, -30.87500000273118772, -5.000000000000000000 ) ) ;
#2399=CARTESIAN_POINT ( 'NONE',  ( 1.846868145590736310, -25.62500000136559564, 4.458734124999999437 ) ) ;
#2406=CARTESIAN_POINT ( 'NONE',  ( 5.000000000000000000, -32.00000000000000000, 0.000000000000000000 ) ) ;
#2407=CARTESIAN_POINT ( 'NONE',  ( -9.184850993605147944E-16, -23.37500000273118772, 5.000000000000000000 ) ) ;
#2409=CARTESIAN_POINT ( 'NONE',  ( -5.000000000000000000, -29.62500000273118417, -6.123233995736766282E-16 ) ) ;
#2411=CARTESIAN_POINT ( 'NONE',  ( 1.846868145590736310, -29.62500000136559208, 4.458734124999997661 ) ) ;
#2415=( BOUNDED_CURVE ( )  B_SPLINE_CURVE ( 2, ( #14804, #11092, #11159, #2422, #15948, #9710, #4872, #9799, #10848 ),
 .UNSPECIFIED., .F., .F. ) 
 B_SPLINE_CURVE_WITH_KNOTS ( ( 3, 2, 2, 2, 3 ),
 ( 0.5250000000000001332, 0.5375000000000000888, 0.5500000000000002665, 0.5625000000000002220, 0.5750000000000001776 ),
 .UNSPECIFIED. ) 
 CURVE ( )  GEOMETRIC_REPRESENTATION_ITEM ( )  RATIONAL_B_SPLINE_CURVE ( ( 0.9999999999999993339, 0.9238795325112874046, 1.000000000000000000, 0.9238795325112867385, 1.000000000000000000, 0.9238795325112867385, 1.000000000000000000, 0.9238795325112854062, 1.000000000000001332 ) ) 
 REPRESENTATION_ITEM ( '' )  );
#2422=CARTESIAN_POINT ( 'NONE',  ( -5.000000000000000888, -25.68750000273118772, -2.071067811865475949 ) ) ;
#2427=CARTESIAN_POINT ( 'NONE',  ( 3.535533905932736864, -24.12500000000000000, 3.535533905932738641 ) ) ;
#2429=MECHANICAL_DESIGN_GEOMETRIC_PRESENTATION_REPRESENTATION('',(#141),#12276);
#2432=SURFACE_STYLE_FILL_AREA ( #13492 ) ;
#2433=VERTEX_POINT ( 'NONE', #2407 ) ;
#2444=CARTESIAN_POINT ( 'NONE',  ( -5.000000000000000888, -30.56250000273118772, 2.071067811865474617 ) ) ;
#2446=CARTESIAN_POINT ( 'NONE',  ( 3.061616997868383141E-16, -24.75000000000000000, -5.000000000000000000 ) ) ;
#2449=CARTESIAN_POINT ( 'NONE',  ( -4.458734125000000326, -24.12500000136559919, 1.846868145590734089 ) ) ;
#2451=CARTESIAN_POINT ( 'NONE',  ( -4.458734124999999437, -21.93750000136559208, -5.460374474430324690E-16 ) ) ;
#2458=CARTESIAN_POINT ( 'NONE',  ( 4.458734125000000326, -24.62500000136559564, -1.846868145590734978 ) ) ;
#2462=DIRECTION ( 'NONE',  ( 0.000000000000000000, -0.000000000000000000, -1.000000000000000000 ) ) ;
#2468=CARTESIAN_POINT ( 'NONE',  ( 4.458734124999999437, -25.43750000136559564, 0.000000000000000000 ) ) ;
#2477=CARTESIAN_POINT ( 'NONE',  ( -4.458734125000001214, -22.87500000136559564, 1.846868145590734089 ) ) ;
#2481=CARTESIAN_POINT ( 'NONE',  ( 4.769696007084728073, -20.00000000000000000, 1.500000000000000000 ) ) ;
#2486=CARTESIAN_POINT ( 'NONE',  ( -4.458734125000001214, -25.12500000136559564, 1.846868145590734089 ) ) ;
#2490=CARTESIAN_POINT ( 'NONE',  ( -3.535533905932737309, -28.75000000273118772, -3.535533905932738197 ) ) ;
#2499=CIRCLE ( 'NONE', #15695, 2.649999999999992806 ) ;
#2501=CARTESIAN_POINT ( 'NONE',  ( 35.00000000000000000, 37.00000000000000000, -8.572527594031472993E-15 ) ) ;
#2523=( GEOMETRIC_REPRESENTATION_CONTEXT ( 3 ) GLOBAL_UNCERTAINTY_ASSIGNED_CONTEXT ( ( #479 ) ) GLOBAL_UNIT_ASSIGNED_CONTEXT ( ( #11657, #14256, #6825 ) ) REPRESENTATION_CONTEXT ( 'NONE', 'WORKASPACE' ) );
#2532=CARTESIAN_POINT ( 'NONE',  ( 4.769696007084728073, -20.00000000000000000, -1.500000000000000000 ) ) ;
#2533=CARTESIAN_POINT ( 'NONE',  ( -8.190561711645485556E-16, -26.93750000136559564, 4.458734124999999437 ) ) ;
#2539=VECTOR ( 'NONE', #13072, 1000.000000000000000 ) ;
#2544=CARTESIAN_POINT ( 'NONE',  ( -3.152801135295367985, -23.06250000136559564, 3.152801135295367096 ) ) ;
#2546=DIRECTION ( 'NONE',  ( -0.000000000000000000, -1.000000000000000000, -0.000000000000000000 ) ) ;
#2551=CARTESIAN_POINT ( 'NONE',  ( 0.000000000000000000, -20.00000000000000000, 5.000000000000000000 ) ) ;
#2556=CARTESIAN_POINT ( 'NONE',  ( 4.458734124999999437, -27.50000000136559208, 1.846868145590737864 ) ) ;
#2563=CARTESIAN_POINT ( 'NONE',  ( 3.152801135295367541, -25.31250000136559564, -3.152801135295367541 ) ) ;
#2568=ADVANCED_FACE ( 'NONE', ( #1447 ), #9219, .T. ) ;
#2574=CARTESIAN_POINT ( 'NONE',  ( -2.071067811865475061, -30.68750000000000355, -5.000000000000000888 ) ) ;
#2577=CARTESIAN_POINT ( 'NONE',  ( -5.000000000000000000, -26.62500000273118772, -6.123233995736766282E-16 ) ) ;
#2578=LINE ( 'NONE', #14966, #353 ) ;
#2579=CARTESIAN_POINT ( 'NONE',  ( 3.152801135295366208, -29.56250000136559208, 3.152801135295367985 ) ) ;
#2595=CARTESIAN_POINT ( 'NONE',  ( 2.071067811865461294, -23.81250000000000000, -5.000000000000014211 ) ) ;
#2606=LINE ( 'NONE', #365, #4522 ) ;
#2608=( BOUNDED_CURVE ( )  B_SPLINE_CURVE ( 2, ( #14735, #9566, #5850, #2120, #14656, #13258, #9635, #14494, #13490 ),
 .UNSPECIFIED., .F., .F. ) 
 B_SPLINE_CURVE_WITH_KNOTS ( ( 3, 2, 2, 2, 3 ),
 ( 0.9250000000000002665, 0.9375000000000002220, 0.9500000000000001776, 0.9625000000000002442, 0.9750000000000001998 ),
 .UNSPECIFIED. ) 
 CURVE ( )  GEOMETRIC_REPRESENTATION_ITEM ( )  RATIONAL_B_SPLINE_CURVE ( ( 0.9999999999999986677, 0.9238795325112880708, 1.000000000000000000, 0.9238795325112867385, 1.000000000000000000, 0.9238795325112867385, 1.000000000000000000, 0.9238795325112854062, 1.000000000000001332 ) ) 
 REPRESENTATION_ITEM ( '' )  );
#2614=CARTESIAN_POINT ( 'NONE',  ( 4.458734124999999437, -31.68750000136559564, 0.000000000000000000 ) ) ;
#2615=CARTESIAN_POINT ( 'NONE',  ( 1.846868145590735200, -25.50000000136559919, -4.458734124999999437 ) ) ;
#2620=EDGE_CURVE ( 'NONE', #11629, #6271, #8818, .T. ) ;
#2627=CARTESIAN_POINT ( 'NONE',  ( -1.846868145590737420, -22.00000000136559208, 4.458734124999999437 ) ) ;
#2629=LINE ( 'NONE', #8869, #12226 ) ;
#2634=CARTESIAN_POINT ( 'NONE',  ( 2.071067811865497710, -30.18750000000000355, 4.999999999999978684 ) ) ;
#2636=CARTESIAN_POINT ( 'NONE',  ( 3.535533905932738197, -28.87500000000000000, -3.535533905932738197 ) ) ;
#2637=CARTESIAN_POINT ( 'NONE',  ( -3.152801135295367985, -24.81250000136559564, 3.152801135295367096 ) ) ;
#2645=CARTESIAN_POINT ( 'NONE',  ( -3.152801135295367985, -25.81250000136559564, 3.152801135295367096 ) ) ;
#2647=ORIENTED_EDGE ( 'NONE', *, *, #3701, .T. ) ;
#2648=AXIS2_PLACEMENT_3D ( 'NONE', #3792, #5089, #15849 ) ;
#2651=DIRECTION ( 'NONE',  ( -1.000000000000000000, 0.000000000000000000, -0.000000000000000000 ) ) ;
#2653=CARTESIAN_POINT ( 'NONE',  ( -5.000000000000000888, -30.43750000000000355, 2.071067811865474617 ) ) ;
#2656=CARTESIAN_POINT ( 'NONE',  ( 2.071067811865475505, -26.93750000273119127, -5.000000000000000888 ) ) ;
#2658=CARTESIAN_POINT ( 'NONE',  ( 4.458734124999997661, -30.50000000136559919, 1.846868145590737864 ) ) ;
#2662=ORIENTED_EDGE ( 'NONE', *, *, #12701, .F. ) ;
#2670=FACE_OUTER_BOUND ( 'NONE', #12081, .T. ) ;
#2694=CARTESIAN_POINT ( 'NONE',  ( -3.535533905932737309, -23.62500000000000000, -3.535533905932738197 ) ) ;
#2695=CARTESIAN_POINT ( 'NONE',  ( 3.535533905932738197, -28.00000000273118772, -3.535533905932738197 ) ) ;
#2708=LINE ( 'NONE', #234, #13017 ) ;
#2716=CARTESIAN_POINT ( 'NONE',  ( 4.458734124999999437, -23.50000000136559564, 1.846868145590737864 ) ) ;
#2725=CARTESIAN_POINT ( 'NONE',  ( 2.730187237215162345E-16, -22.18750000136559564, -4.458734124999999437 ) ) ;
#2727=ORIENTED_EDGE ( 'NONE', *, *, #13000, .F. ) ;
#2729=AXIS2_PLACEMENT_3D ( 'NONE', #4100, #8077, #481 ) ;
#2736=CARTESIAN_POINT ( 'NONE',  ( 2.071067811865476394, -28.18750000000000711, 5.000000000000000000 ) ) ;
#2739=CARTESIAN_POINT ( 'NONE',  ( -5.000000000000000888, -27.68750000273119127, -2.071067811865475949 ) ) ;
#2740=DIRECTION ( 'NONE',  ( 0.8660254037844410391, 0.4999999999999958367, -0.000000000000000000 ) ) ;
#2741=CARTESIAN_POINT ( 'NONE',  ( -8.190561711645485556E-16, -29.68750000136559208, 4.458734124999999437 ) ) ;
#2754=CARTESIAN_POINT ( 'NONE',  ( -5.000000000000000888, -31.56250000000000000, -2.071067811865475949 ) ) ;
#2756=LINE ( 'NONE', #7623, #10042 ) ;
#2774=CARTESIAN_POINT ( 'NONE',  ( -2.071067811865492381, -28.43750000273118772, 4.999999999999985789 ) ) ;
#2779=CARTESIAN_POINT ( 'NONE',  ( 0.000000000000000000, -11.00000000000000178, -6.000000000000000888 ) ) ;
#2782=DIRECTION ( 'NONE',  ( -0.000000000000000000, -1.000000000000000000, -0.000000000000000000 ) ) ;
#2783=VERTEX_POINT ( 'NONE', #9372 ) ;
#2784=DIRECTION ( 'NONE',  ( 0.000000000000000000, 0.000000000000000000, 1.000000000000000000 ) ) ;
#2788=ORIENTED_EDGE ( 'NONE', *, *, #13644, .F. ) ;
#2798=CARTESIAN_POINT ( 'NONE',  ( 0.000000000000000000, -13.00000000000000178, -1.500000000000000000 ) ) ;
#2803=AXIS2_PLACEMENT_3D ( 'NONE', #10401, #5394, #6929 ) ;
#2805=CARTESIAN_POINT ( 'NONE',  ( -4.458734125000001214, -21.87500000136559208, 1.846868145590734089 ) ) ;
#2806=AXIS2_PLACEMENT_3D ( 'NONE', #9851, #15693, #4925 ) ;
#2810=VERTEX_POINT ( 'NONE', #5801 ) ;
#2812=CARTESIAN_POINT ( 'NONE',  ( 1.846868145590735200, -30.50000000136559919, -4.458734125000000326 ) ) ;
#2820=CARTESIAN_POINT ( 'NONE',  ( -35.00000000000000000, 40.00000000000000000, 0.000000000000000000 ) ) ;
#2821=CARTESIAN_POINT ( 'NONE',  ( -5.000000000000000888, -29.43750000000000711, 2.071067811865474617 ) ) ;
#2824=CARTESIAN_POINT ( 'NONE',  ( -5.000000000000000888, -22.68750000273119127, -2.071067811865475949 ) ) ;
#2826=CARTESIAN_POINT ( 'NONE',  ( -1.846868145590734756, -26.12500000136559564, -4.458734124999999437 ) ) ;
#2828=ORIENTED_EDGE ( 'NONE', *, *, #15232, .F. ) ;
#2829=ORIENTED_EDGE ( 'NONE', *, *, #12086, .F. ) ;
#2832=ORIENTED_EDGE ( 'NONE', *, *, #4447, .F. ) ;
#2838=CARTESIAN_POINT ( 'NONE',  ( -8.190561711645485556E-16, -29.93750000136559564, 4.458734124999999437 ) ) ;
#2845=CARTESIAN_POINT ( 'NONE',  ( -4.458734125000000326, -31.00000000136559564, -1.846868145590735644 ) ) ;
#2855=FILL_AREA_STYLE ('',( #7968 ) ) ;
#2856=CARTESIAN_POINT ( 'NONE',  ( -4.458734124999999437, -22.25000000136559564, -1.846868145590735644 ) ) ;
#2866=EDGE_CURVE ( 'NONE', #8315, #3368, #12331, .T. ) ;
#2869=CARTESIAN_POINT ( 'NONE',  ( 6.123233995736766282E-16, -20.00000000000000000, -5.000000000000000000 ) ) ;
#2878=FACE_OUTER_BOUND ( 'NONE', #15227, .T. ) ;
#2879=CARTESIAN_POINT ( 'NONE',  ( 0.000000000000000000, -20.00000000000000000, -1.500000000000000000 ) ) ;
#2880=CARTESIAN_POINT ( 'NONE',  ( -8.190561711645485556E-16, -23.68750000136559564, 4.458734124999999437 ) ) ;
#2889=CARTESIAN_POINT ( 'NONE',  ( -4.458734125000000326, -29.25000000136559564, -1.846868145590735644 ) ) ;
#2891=ORIENTED_EDGE ( 'NONE', *, *, #8811, .F. ) ;
#2895=LINE ( 'NONE', #12742, #12713 ) ;
#2896=CARTESIAN_POINT ( 'NONE',  ( -2.071067811865478170, -30.31249999999999645, 5.000000000000000000 ) ) ;
#2900=CARTESIAN_POINT ( 'NONE',  ( 3.535533905932736864, -26.25000000273118417, 3.535533905932738641 ) ) ;
#2902=CARTESIAN_POINT ( 'NONE',  ( 2.730187237215162345E-16, -25.18750000136559564, -4.458734124999999437 ) ) ;
#2907=AXIS2_PLACEMENT_3D ( 'NONE', #14848, #8558, #3768 ) ;
#2912=DIRECTION ( 'NONE',  ( 0.000000000000000000, 0.000000000000000000, 1.000000000000000000 ) ) ;
#2913=CARTESIAN_POINT ( 'NONE',  ( 3.152801135295366208, -29.81250000136559208, 3.152801135295367985 ) ) ;
#2923=CARTESIAN_POINT ( 'NONE',  ( 1.846868145590736310, -28.62500000136559919, 4.458734124999999437 ) ) ;
#2929=EDGE_CURVE ( 'NONE', #3228, #10093, #2390, .T. ) ;
#2931=CARTESIAN_POINT ( 'NONE',  ( 0.000000000000000000, -32.00000000000000000, 5.000000000000000000 ) ) ;
#2933=CARTESIAN_POINT ( 'NONE',  ( -1.846868145590737420, -23.00000000136559564, 4.458734124999997661 ) ) ;
#2940=ORIENTED_EDGE ( 'NONE', *, *, #335, .T. ) ;
#2941=( BOUNDED_SURFACE ( )  B_SPLINE_SURFACE ( 1, 2, ( 
 ( #4132, #11481, #12443, #1377, #12523, #11244, #5108, #7712, #13660, #10044, #14977, #13983, #10367, #1467, #15297, #8999, #1625, #274, #5191, #428, #1550, #5353, #12608, #13911, #10291, #15052, #6653, #3966, #2838, #7789, #2913, #7864, #12762, #11562, #10760, #6806, #5591, #747, #5744, #13003, #14163, #5672, #10439, #10680, #901, #15376, #12848, #10610, #9237, #3092, #15611, #14398, #10528, #4453, #4532, #15538, #11951, #11637, #4210, #9466, #4298, #2999, #5823, #9155, #9317, #9388, #3325, #14312, #8276, #3241, #11875, #8188, #11711, #14238, #3160, #8032, #14072, #13167, #2027, #2103, #13088, #6890, #666, #11794, #6974, #1790, #821, #7047, #7949, #6735, #588, #5511, #12925, #1860, #15463, #4383, #8109, #1942, #3708, #11, #1207, #4928, #1123, #8655, #13553, #2486, #8344, #12184, #9612, #2339, #3635, #12354, #7128, #9856, #7447, #1286, #12266, #12030, #2177, #14548, #6231, #14787, #6152, #15697, #6063, #4613, #9546, #14473, #13240, #10992, #3468, #5984, #3395, #980, #5911, #10836, #15776, #4687, #7358, #14712, #8427, #13316, #13401, #15931, #2259, #7282, #7212, #4854, #12114, #1050, #11079, #13468, #10908, #15850, #4768, #9692, #14631, #3549, #8506, #9780, #8579 ),
 ( #2406, #8819, #7775, #13720, #6310, #6391, #15199, #9062, #6472, #11310, #1446, #15107, #5175, #4114, #13645, #11145, #11227, #5090, #5249, #10185, #172, #2574, #11462, #13964, #10025, #2653, #87, #2896, #5004, #7525, #11384, #10271, #1534, #12590, #3950, #8979, #3877, #7846, #336, #8739, #12744, #2821, #8895, #12666, #7604, #1688, #5333, #409, #260, #9932, #4027, #10104, #13891, #14961, #12503, #14871, #3793, #15036, #12428, #1361, #13798, #2736, #7692, #1606, #6547, #649, #10595, #10350, #11694, #6629, #14049, #9137, #570, #10659, #6956, #8166, #11857, #8090, #15592, #4511, #9446, #15277, #3143, #5491, #12908, #8257, #3303, #11542, #14376, #13149, #804, #14295, #5654, #494, #1770, #4365, #12984, #6717, #9299, #11620, #1920, #4191, #5418, #13068, #4435, #2975, #7929, #10421, #12826, #15356, #5572, #4275, #9217, #14139, #5724, #3069, #8012, #1843, #6868, #15519, #6786, #10509, #3218, #15443, #9370, #14222, #11775, #2006, #728, #3525, #9593, #8401, #1102, #12007, #7337, #9527, #6042, #8635, #4669, #3448, #14605, #3614, #10887, #959, #3526, #8328, #8559, #14766, #13218, #10737, #8480, #7106, #5884, #13448, #12242, #13292, #2319, #2388, #13381, #9834, #14456 ) ),
 .UNSPECIFIED., .F., .F., .F. ) 
 B_SPLINE_SURFACE_WITH_KNOTS ( ( 2, 2 ),
 ( 3, 2, 2, 2, 2, 2, 2, 2, 2, 2, 2, 2, 2, 2, 2, 2, 2, 2, 2, 2, 2, 2, 2, 2, 2, 2, 2, 2, 2, 2, 2, 2, 2, 2, 2, 2, 2, 2, 2, 2, 2, 2, 2, 2, 2, 2, 2, 2, 2, 2, 2, 2, 2, 2, 2, 2, 2, 2, 2, 2, 2, 2, 2, 2, 2, 2, 2, 2, 2, 2, 2, 2, 2, 2, 2, 2, 2, 2, 2, 2, 3 ),
 ( 0.000000000000000000, 1.000000000000000000 ),
 ( 0.000000000000000000, 0.01250000000000000069, 0.02500000000000000139, 0.03749999999999999861, 0.05000000000000000278, 0.06250000000000000000, 0.07499999999999999722, 0.08749999999999999445, 0.1000000000000000056, 0.1125000000000000028, 0.1250000000000000000, 0.1375000000000000111, 0.1499999999999999944, 0.1625000000000000056, 0.1749999999999999889, 0.1875000000000000000, 0.2000000000000000111, 0.2124999999999999944, 0.2250000000000000056, 0.2374999999999999889, 0.2500000000000000000, 0.2625000000000000111, 0.2750000000000000222, 0.2874999999999999778, 0.2999999999999999889, 0.3125000000000000000, 0.3250000000000000111, 0.3375000000000000222, 0.3499999999999999778, 0.3624999999999999889, 0.3750000000000000000, 0.3875000000000000111, 0.4000000000000000222, 0.4124999999999999778, 0.4249999999999999889, 0.4375000000000000000, 0.4500000000000000111, 0.4625000000000000222, 0.4749999999999999778, 0.4874999999999999889, 0.5000000000000000000, 0.5124999999999999556, 0.5250000000000000222, 0.5374999999999999778, 0.5500000000000000444, 0.5625000000000000000, 0.5749999999999999556, 0.5875000000000000222, 0.5999999999999999778, 0.6125000000000000444, 0.6250000000000000000, 0.6374999999999999556, 0.6500000000000000222, 0.6624999999999999778, 0.6750000000000000444, 0.6875000000000000000, 0.6999999999999999556, 0.7125000000000000222, 0.7249999999999999778, 0.7375000000000000444, 0.7500000000000000000, 0.7624999999999999556, 0.7750000000000000222, 0.7874999999999999778, 0.8000000000000000444, 0.8125000000000000000, 0.8249999999999999556, 0.8375000000000000222, 0.8499999999999999778, 0.8625000000000000444, 0.8750000000000000000, 0.8874999999999999556, 0.9000000000000000222, 0.9124999999999999778, 0.9250000000000000444, 0.9375000000000000000, 0.9499999999999999556, 0.9625000000000000222, 0.9749999999999999778, 0.9875000000000000444, 1.000000000000000000 ),
 .UNSPECIFIED. ) 
 GEOMETRIC_REPRESENTATION_ITEM ( )  RATIONAL_B_SPLINE_SURFACE ( (
 ( 1.000000000000000000, 0.9238795325112867385, 1.000000000000000000, 0.9238795325112867385, 1.000000000000000000, 0.9238795325112867385, 1.000000000000000000, 0.9238795325112867385, 1.000000000000000000, 0.9238795325112867385, 1.000000000000000000, 0.9238795325112867385, 1.000000000000000000, 0.9238795325112867385, 1.000000000000000000, 0.9238795325112867385, 1.000000000000000000, 0.9238795325112867385, 1.000000000000000000, 0.9238795325112867385, 1.000000000000000000, 0.9238795325112867385, 1.000000000000000000, 0.9238795325112867385, 1.000000000000000000, 0.9238795325112867385, 1.000000000000000000, 0.9238795325112867385, 1.000000000000000000, 0.9238795325112867385, 1.000000000000000000, 0.9238795325112867385, 1.000000000000000000, 0.9238795325112867385, 1.000000000000000000, 0.9238795325112867385, 1.000000000000000000, 0.9238795325112867385, 1.000000000000000000, 0.9238795325112867385, 1.000000000000000000, 0.9238795325112867385, 1.000000000000000000, 0.9238795325112867385, 1.000000000000000000, 0.9238795325112867385, 1.000000000000000000, 0.9238795325112867385, 1.000000000000000000, 0.9238795325112867385, 1.000000000000000000, 0.9238795325112867385, 1.000000000000000000, 0.9238795325112867385, 1.000000000000000000, 0.9238795325112867385, 1.000000000000000000, 0.9238795325112867385, 1.000000000000000000, 0.9238795325112867385, 1.000000000000000000, 0.9238795325112867385, 1.000000000000000000, 0.9238795325112867385, 1.000000000000000000, 0.9238795325112867385, 1.000000000000000000, 0.9238795325112867385, 1.000000000000000000, 0.9238795325112867385, 1.000000000000000000, 0.9238795325112867385, 1.000000000000000000, 0.9238795325112867385, 1.000000000000000000, 0.9238795325112867385, 1.000000000000000000, 0.9238795325112867385, 1.000000000000000000, 0.9238795325112867385, 1.000000000000000000, 0.9238795325112867385, 1.000000000000000000, 0.9238795325112867385, 1.000000000000000000, 0.9238795325112867385, 1.000000000000000000, 0.9238795325112867385, 1.000000000000000000, 0.9238795325112867385, 1.000000000000000000, 0.9238795325112867385, 1.000000000000000000, 0.9238795325112867385, 1.000000000000000000, 0.9238795325112867385, 1.000000000000000000, 0.9238795325112867385, 1.000000000000000000, 0.9238795325112867385, 1.000000000000000000, 0.9238795325112867385, 1.000000000000000000, 0.9238795325112867385, 1.000000000000000000, 0.9238795325112867385, 1.000000000000000000, 0.9238795325112867385, 1.000000000000000000, 0.9238795325112867385, 1.000000000000000000, 0.9238795325112867385, 1.000000000000000000, 0.9238795325112867385, 1.000000000000000000, 0.9238795325112867385, 1.000000000000000000, 0.9238795325112867385, 1.000000000000000000, 0.9238795325112867385, 1.000000000000000000, 0.9238795325112867385, 1.000000000000000000, 0.9238795325112867385, 1.000000000000000000, 0.9238795325112867385, 1.000000000000000000, 0.9238795325112867385, 1.000000000000000000, 0.9238795325112867385, 1.000000000000000000, 0.9238795325112867385, 1.000000000000000000, 0.9238795325112867385, 1.000000000000000000, 0.9238795325112867385, 1.000000000000000000, 0.9238795325112867385, 1.000000000000000000, 0.9238795325112867385, 1.000000000000000000, 0.9238795325112867385, 1.000000000000000000, 0.9238795325112867385, 1.000000000000000000, 0.9238795325112867385, 1.000000000000000000, 0.9238795325112867385, 1.000000000000000000, 0.9238795325112867385, 1.000000000000000000, 0.9238795325112867385, 1.000000000000000000, 0.9238795325112867385, 1.000000000000000000, 0.9238795325112867385, 1.000000000000000000, 0.9238795325112867385, 1.000000000000000000, 0.9238795325112867385, 1.000000000000000000),
 ( 1.000000000000000000, 0.9238795325112867385, 1.000000000000000000, 0.9238795325112867385, 1.000000000000000000, 0.9238795325112867385, 1.000000000000000000, 0.9238795325112867385, 1.000000000000000000, 0.9238795325112867385, 1.000000000000000000, 0.9238795325112867385, 1.000000000000000000, 0.9238795325112867385, 1.000000000000000000, 0.9238795325112867385, 1.000000000000000000, 0.9238795325112867385, 1.000000000000000000, 0.9238795325112867385, 1.000000000000000000, 0.9238795325112867385, 1.000000000000000000, 0.9238795325112867385, 1.000000000000000000, 0.9238795325112867385, 1.000000000000000000, 0.9238795325112867385, 1.000000000000000000, 0.9238795325112867385, 1.000000000000000000, 0.9238795325112867385, 1.000000000000000000, 0.9238795325112867385, 1.000000000000000000, 0.9238795325112867385, 1.000000000000000000, 0.9238795325112867385, 1.000000000000000000, 0.9238795325112867385, 1.000000000000000000, 0.9238795325112867385, 1.000000000000000000, 0.9238795325112867385, 1.000000000000000000, 0.9238795325112867385, 1.000000000000000000, 0.9238795325112867385, 1.000000000000000000, 0.9238795325112867385, 1.000000000000000000, 0.9238795325112867385, 1.000000000000000000, 0.9238795325112867385, 1.000000000000000000, 0.9238795325112867385, 1.000000000000000000, 0.9238795325112867385, 1.000000000000000000, 0.9238795325112867385, 1.000000000000000000, 0.9238795325112867385, 1.000000000000000000, 0.9238795325112867385, 1.000000000000000000, 0.9238795325112867385, 1.000000000000000000, 0.9238795325112867385, 1.000000000000000000, 0.9238795325112867385, 1.000000000000000000, 0.9238795325112867385, 1.000000000000000000, 0.9238795325112867385, 1.000000000000000000, 0.9238795325112867385, 1.000000000000000000, 0.9238795325112867385, 1.000000000000000000, 0.9238795325112867385, 1.000000000000000000, 0.9238795325112867385, 1.000000000000000000, 0.9238795325112867385, 1.000000000000000000, 0.9238795325112867385, 1.000000000000000000, 0.9238795325112867385, 1.000000000000000000, 0.9238795325112867385, 1.000000000000000000, 0.9238795325112867385, 1.000000000000000000, 0.9238795325112867385, 1.000000000000000000, 0.9238795325112867385, 1.000000000000000000, 0.9238795325112867385, 1.000000000000000000, 0.9238795325112867385, 1.000000000000000000, 0.9238795325112867385, 1.000000000000000000, 0.9238795325112867385, 1.000000000000000000, 0.9238795325112867385, 1.000000000000000000, 0.9238795325112867385, 1.000000000000000000, 0.9238795325112867385, 1.000000000000000000, 0.9238795325112867385, 1.000000000000000000, 0.9238795325112867385, 1.000000000000000000, 0.9238795325112867385, 1.000000000000000000, 0.9238795325112867385, 1.000000000000000000, 0.9238795325112867385, 1.000000000000000000, 0.9238795325112867385, 1.000000000000000000, 0.9238795325112867385, 1.000000000000000000, 0.9238795325112867385, 1.000000000000000000, 0.9238795325112867385, 1.000000000000000000, 0.9238795325112867385, 1.000000000000000000, 0.9238795325112867385, 1.000000000000000000, 0.9238795325112867385, 1.000000000000000000, 0.9238795325112867385, 1.000000000000000000, 0.9238795325112867385, 1.000000000000000000, 0.9238795325112867385, 1.000000000000000000, 0.9238795325112867385, 1.000000000000000000, 0.9238795325112867385, 1.000000000000000000, 0.9238795325112867385, 1.000000000000000000, 0.9238795325112867385, 1.000000000000000000, 0.9238795325112867385, 1.000000000000000000, 0.9238795325112867385, 1.000000000000000000, 0.9238795325112867385, 1.000000000000000000, 0.9238795325112867385, 1.000000000000000000, 0.9238795325112867385, 1.000000000000000000, 0.9238795325112867385, 1.000000000000000000) ) ) 
 REPRESENTATION_ITEM ( '' )  SURFACE ( )  );
#2949=CARTESIAN_POINT ( 'NONE',  ( 5.000000000000000000, -26.18750000273118772, 2.071067811865478614 ) ) ;
#2951=ADVANCED_FACE ( 'NONE', ( #2878 ), #11603, .T. ) ;
#2955=CARTESIAN_POINT ( 'NONE',  ( -9.184850993605147944E-16, -30.25000000000000000, 5.000000000000000000 ) ) ;
#2957=CARTESIAN_POINT ( 'NONE',  ( 4.458734124999999437, -24.43750000136559564, 0.000000000000000000 ) ) ;
#2966=CARTESIAN_POINT ( 'NONE',  ( -1.846868145590734756, -30.37500000136559564, -4.458734125000000326 ) ) ;
#2974=EDGE_CURVE ( 'NONE', #3368, #8728, #10973, .T. ) ;
#2975=CARTESIAN_POINT ( 'NONE',  ( -5.000000000000000888, -25.43750000000000355, 2.071067811865474617 ) ) ;
#2976=CIRCLE ( 'NONE', #8422, 25.00000000000000000 ) ;
#2980=CARTESIAN_POINT ( 'NONE',  ( -2.071067811865478170, -23.43750000273119127, 5.000000000000000000 ) ) ;
#2981=CIRCLE ( 'NONE', #1434, 6.000000000000000888 ) ;
#2982=CARTESIAN_POINT ( 'NONE',  ( 4.729367062499999719, -21.28125000204839168, 0.000000000000000000 ) ) ;
#2984=CARTESIAN_POINT ( 'NONE',  ( -3.152801135295367096, -25.06250000136559564, -3.152801135295367541 ) ) ;
#2989=VERTEX_POINT ( 'NONE', #15260 ) ;
#2999=CARTESIAN_POINT ( 'NONE',  ( 1.846868145590736310, -27.87500000136559564, 4.458734124999999437 ) ) ;
#3002=PLANE ( 'NONE',  #12312 ) ;
#3003=CARTESIAN_POINT ( 'NONE',  ( 5.000000000000000000, -31.12500000273118772, 0.000000000000000000 ) ) ;
#3009=CARTESIAN_POINT ( 'NONE',  ( 3.152801135295367541, -30.31250000136559564, -3.152801135295367541 ) ) ;
#3010=ORIENTED_EDGE ( 'NONE', *, *, #13000, .T. ) ;
#3016=DIRECTION ( 'NONE',  ( 0.000000000000000000, 0.000000000000000000, 1.000000000000000000 ) ) ;
#3024=DIRECTION ( 'NONE',  ( 0.000000000000000000, 0.000000000000000000, 1.000000000000000000 ) ) ;
#3026=CARTESIAN_POINT ( 'NONE',  ( -3.535533905932737309, -26.75000000273118772, -3.535533905932738197 ) ) ;
#3047=CARTESIAN_POINT ( 'NONE',  ( -4.458734124999999437, -23.93750000136559564, -5.460374474430324690E-16 ) ) ;
#3048=( BOUNDED_CURVE ( )  B_SPLINE_CURVE ( 2, ( #7088, #9283, #13276, #6936, #5710, #5869, #8235, #9580, #15504, #3129, #4496, #8313, #940, #9509, #3365, #7172, #4654, #8386, #10722, #11990, #5636, #9431, #15579, #3432, #14359, #5951, #10802, #13202, #2141, #3288, #15656, #15742, #14205, #2218, #11841, #13133, #14511, #2069, #12074, #4420, #8073, #12969, #1018, #15423, #4574, #4345, #9355, #7013, #1904, #788, #6850, #14441, #14280, #11915, #11757, #711, #10579, #3202, #8151, #13048, #1988, #863, #5783, #9980, #13511, #7487, #10871, #12151, #3508, #1248, #4814, #7405, #14919, #12309, #5050, #6196, #2533, #9894, #2374, #11524, #4895, #13365, #1088, #15893, #7251, #14831, #4967, #51, #8466, #11113, #3839, #13434, #1165, #8546, #8782, #2306, #1405, #6028, #9820, #2615, #13684, #10950, #7569, #9736, #3672, #3750, #12466, #8698, #7322, #14587, #15813, #14674, #13601, #3599, #6109, #4730, #9651, #12224, #11036, #14749, #8619, #2449, #12390, #1326, #6270, #11184, #129, #9177, #15318, #11425, #453, #12873, #11270, #11586, #5375, #6678, #538, #15070, #12551, #2933, #10231, #13930, #15243, #12631, #10317, #3912, #4152, #12783, #9098, #6351, #14099, #2856, #7811, #5455, #6511, #218, #1646, #372, #11501, #5211, #10146 ),
 .UNSPECIFIED., .F., .F. ) 
 B_SPLINE_CURVE_WITH_KNOTS ( ( 3, 2, 2, 2, 2, 2, 2, 2, 2, 2, 2, 2, 2, 2, 2, 2, 2, 2, 2, 2, 2, 2, 2, 2, 2, 2, 2, 2, 2, 2, 2, 2, 2, 2, 2, 2, 2, 2, 2, 2, 2, 2, 2, 2, 2, 2, 2, 2, 2, 2, 2, 2, 2, 2, 2, 2, 2, 2, 2, 2, 2, 2, 2, 2, 2, 2, 2, 2, 2, 2, 2, 2, 2, 2, 2, 2, 2, 2, 2, 2, 3 ),
 ( 0.000000000000000000, 0.01250000000000000069, 0.02500000000000000139, 0.03749999999999999861, 0.05000000000000000278, 0.06250000000000000000, 0.07499999999999999722, 0.08749999999999999445, 0.1000000000000000056, 0.1125000000000000028, 0.1250000000000000000, 0.1375000000000000111, 0.1499999999999999944, 0.1625000000000000056, 0.1749999999999999889, 0.1875000000000000000, 0.2000000000000000111, 0.2124999999999999944, 0.2250000000000000056, 0.2374999999999999889, 0.2500000000000000000, 0.2625000000000000111, 0.2750000000000000222, 0.2874999999999999778, 0.2999999999999999889, 0.3125000000000000000, 0.3250000000000000111, 0.3375000000000000222, 0.3499999999999999778, 0.3624999999999999889, 0.3750000000000000000, 0.3875000000000000111, 0.4000000000000000222, 0.4124999999999999778, 0.4249999999999999889, 0.4375000000000000000, 0.4500000000000000111, 0.4625000000000000222, 0.4749999999999999778, 0.4874999999999999889, 0.5000000000000000000, 0.5124999999999999556, 0.5250000000000000222, 0.5374999999999999778, 0.5500000000000000444, 0.5625000000000000000, 0.5749999999999999556, 0.5875000000000000222, 0.5999999999999999778, 0.6125000000000000444, 0.6250000000000000000, 0.6374999999999999556, 0.6500000000000000222, 0.6624999999999999778, 0.6750000000000000444, 0.6875000000000000000, 0.6999999999999999556, 0.7125000000000000222, 0.7249999999999999778, 0.7375000000000000444, 0.7500000000000000000, 0.7624999999999999556, 0.7750000000000000222, 0.7874999999999999778, 0.8000000000000000444, 0.8125000000000000000, 0.8249999999999999556, 0.8375000000000000222, 0.8499999999999999778, 0.8625000000000000444, 0.8750000000000000000, 0.8874999999999999556, 0.9000000000000000222, 0.9124999999999999778, 0.9250000000000000444, 0.9375000000000000000, 0.9499999999999999556, 0.9625000000000000222, 0.9749999999999999778, 0.9875000000000000444, 1.000000000000000000 ),
 .UNSPECIFIED. ) 
 CURVE ( )  GEOMETRIC_REPRESENTATION_ITEM ( )  RATIONAL_B_SPLINE_CURVE ( ( 1.000000000000000000, 0.9238795325112867385, 1.000000000000000000, 0.9238795325112867385, 1.000000000000000000, 0.9238795325112867385, 1.000000000000000000, 0.9238795325112867385, 1.000000000000000000, 0.9238795325112867385, 1.000000000000000000, 0.9238795325112867385, 1.000000000000000000, 0.9238795325112867385, 1.000000000000000000, 0.9238795325112867385, 1.000000000000000000, 0.9238795325112867385, 1.000000000000000000, 0.9238795325112867385, 1.000000000000000000, 0.9238795325112867385, 1.000000000000000000, 0.9238795325112867385, 1.000000000000000000, 0.9238795325112867385, 1.000000000000000000, 0.9238795325112867385, 1.000000000000000000, 0.9238795325112867385, 1.000000000000000000, 0.9238795325112867385, 1.000000000000000000, 0.9238795325112867385, 1.000000000000000000, 0.9238795325112867385, 1.000000000000000000, 0.9238795325112867385, 1.000000000000000000, 0.9238795325112867385, 1.000000000000000000, 0.9238795325112867385, 1.000000000000000000, 0.9238795325112867385, 1.000000000000000000, 0.9238795325112867385, 1.000000000000000000, 0.9238795325112867385, 1.000000000000000000, 0.9238795325112867385, 1.000000000000000000, 0.9238795325112867385, 1.000000000000000000, 0.9238795325112867385, 1.000000000000000000, 0.9238795325112867385, 1.000000000000000000, 0.9238795325112867385, 1.000000000000000000, 0.9238795325112867385, 1.000000000000000000, 0.9238795325112867385, 1.000000000000000000, 0.9238795325112867385, 1.000000000000000000, 0.9238795325112867385, 1.000000000000000000, 0.9238795325112867385, 1.000000000000000000, 0.9238795325112867385, 1.000000000000000000, 0.9238795325112867385, 1.000000000000000000, 0.9238795325112867385, 1.000000000000000000, 0.9238795325112867385, 1.000000000000000000, 0.9238795325112867385, 1.000000000000000000, 0.9238795325112867385, 1.000000000000000000, 0.9238795325112867385, 1.000000000000000000, 0.9238795325112867385, 1.000000000000000000, 0.9238795325112867385, 1.000000000000000000, 0.9238795325112867385, 1.000000000000000000, 0.9238795325112867385, 1.000000000000000000, 0.9238795325112867385, 1.000000000000000000, 0.9238795325112867385, 1.000000000000000000, 0.9238795325112867385, 1.000000000000000000, 0.9238795325112867385, 1.000000000000000000, 0.9238795325112867385, 1.000000000000000000, 0.9238795325112867385, 1.000000000000000000, 0.9238795325112867385, 1.000000000000000000, 0.9238795325112867385, 1.000000000000000000, 0.9238795325112867385, 1.000000000000000000, 0.9238795325112867385, 1.000000000000000000, 0.9238795325112867385, 1.000000000000000000, 0.9238795325112867385, 1.000000000000000000, 0.9238795325112867385, 1.000000000000000000, 0.9238795325112867385, 1.000000000000000000, 0.9238795325112867385, 1.000000000000000000, 0.9238795325112867385, 1.000000000000000000, 0.9238795325112867385, 1.000000000000000000, 0.9238795325112867385, 1.000000000000000000, 0.9238795325112867385, 1.000000000000000000, 0.9238795325112867385, 1.000000000000000000, 0.9238795325112867385, 1.000000000000000000, 0.9238795325112867385, 1.000000000000000000, 0.9238795325112867385, 1.000000000000000000, 0.9238795325112867385, 1.000000000000000000, 0.9238795325112867385, 1.000000000000000000, 0.9238795325112867385, 1.000000000000000000, 0.9238795325112867385, 1.000000000000000000, 0.9238795325112867385, 1.000000000000000000, 0.9238795325112867385, 1.000000000000000000, 0.9238795325112867385, 1.000000000000000000, 0.9238795325112867385, 1.000000000000000000, 0.9238795325112867385, 1.000000000000000000, 0.9238795325112867385, 1.000000000000000000, 0.9238795325112867385, 1.000000000000000000, 0.9238795325112867385, 1.000000000000000000 ) ) 
 REPRESENTATION_ITEM ( '' )  );
#3058=CARTESIAN_POINT ( 'NONE',  ( 4.458734125000000326, -29.62500000136559208, -1.846868145590734978 ) ) ;
#3069=CARTESIAN_POINT ( 'NONE',  ( 2.071067811865475505, -24.81250000000000000, -5.000000000000000888 ) ) ;
#3073=CARTESIAN_POINT ( 'NONE',  ( -2.071067811865478170, -25.43750000273118772, 5.000000000000000000 ) ) ;
#3076=CARTESIAN_POINT ( 'NONE',  ( -3.152801135295367985, -27.81250000136559564, 3.152801135295367096 ) ) ;
#3081=ORIENTED_EDGE ( 'NONE', *, *, #4447, .T. ) ;
#3089=ORIENTED_EDGE ( 'NONE', *, *, #5802, .F. ) ;
#3092=CARTESIAN_POINT ( 'NONE',  ( 4.458734125000000326, -28.62500000136559919, -1.846868145590734978 ) ) ;
#3117=ORIENTED_EDGE ( 'NONE', *, *, #15732, .T. ) ;
#3123=CARTESIAN_POINT ( 'NONE',  ( -3.535533905932737309, -25.62500000000000355, -3.535533905932738197 ) ) ;
#3124=CARTESIAN_POINT ( 'NONE',  ( -9.184850993605147944E-16, -26.25000000000000355, 5.000000000000000000 ) ) ;
#3128=EDGE_CURVE ( 'NONE', #11629, #13499, #4252, .T. ) ;
#3129=CARTESIAN_POINT ( 'NONE',  ( -4.458734125000000326, -31.12500000136559564, 1.846868145590734089 ) ) ;
#3135=CARTESIAN_POINT ( 'NONE',  ( -1.846868145590737420, -27.00000000136559208, 4.458734124999999437 ) ) ;
#3143=CARTESIAN_POINT ( 'NONE',  ( 3.535533905932738197, -26.87500000000000000, -3.535533905932738197 ) ) ;
#3148=EDGE_CURVE ( 'NONE', #8470, #3419, #12891, .T. ) ;
#3149=CARTESIAN_POINT ( 'NONE',  ( -3.535533905932737309, -24.75000000273118417, -3.535533905932738197 ) ) ;
#3151=CARTESIAN_POINT ( 'NONE',  ( -3.152801135295367985, -25.81250000136559564, 3.152801135295367096 ) ) ;
#3154=VERTEX_POINT ( 'NONE', #4343 ) ;
#3157=VERTEX_POINT ( 'NONE', #2139 ) ;
#3158=CARTESIAN_POINT ( 'NONE',  ( 3.061616997868383141E-16, -30.75000000000000000, -5.000000000000000000 ) ) ;
#3160=CARTESIAN_POINT ( 'NONE',  ( -3.152801135295367985, -27.06250000136559564, 3.152801135295367096 ) ) ;
#3166=CIRCLE ( 'NONE', #2648, 6.000000000000000888 ) ;
#3177=CIRCLE ( 'NONE', #13737, 5.999999999999991118 ) ;
#3182=VECTOR ( 'NONE', #7339, 1000.000000000000000 ) ;
#3202=CARTESIAN_POINT ( 'NONE',  ( -4.458734125000000326, -28.12500000136559564, 1.846868145590734089 ) ) ;
#3209=CARTESIAN_POINT ( 'NONE',  ( 4.458734124999999437, -27.68750000136559564, 0.000000000000000000 ) ) ;
#3213=EDGE_CURVE ( 'NONE', #4719, #4136, #14277, .T. ) ;
#3218=CARTESIAN_POINT ( 'NONE',  ( -3.535533905932738641, -24.37500000000000000, 3.535533905932737309 ) ) ;
#3222=CARTESIAN_POINT ( 'NONE',  ( 2.730187237215162345E-16, -29.18750000136559208, -4.458734124999999437 ) ) ;
#3223=AXIS2_PLACEMENT_3D ( 'NONE', #11897, #11972, #4638 ) ;
#3224=ORIENTED_EDGE ( 'NONE', *, *, #1439, .T. ) ;
#3226=CYLINDRICAL_SURFACE ( 'NONE', #1487, 5.000000000000000000 ) ;
#3228=VERTEX_POINT ( 'NONE', #14203 ) ;
#3237=( BOUNDED_CURVE ( )  B_SPLINE_CURVE ( 2, ( #10790, #11667, #3274, #4485, #5543, #14268, #11978, #12883, #10475 ),
 .UNSPECIFIED., .F., .F. ) 
 B_SPLINE_CURVE_WITH_KNOTS ( ( 3, 2, 2, 2, 3 ),
 ( 0.1250000000000001110, 0.1375000000000001221, 0.1500000000000001332, 0.1625000000000001443, 0.1750000000000001554 ),
 .UNSPECIFIED. ) 
 CURVE ( )  GEOMETRIC_REPRESENTATION_ITEM ( )  RATIONAL_B_SPLINE_CURVE ( ( 0.9999999999999993339, 0.9238795325112874046, 1.000000000000000000, 0.9238795325112867385, 1.000000000000000000, 0.9238795325112867385, 1.000000000000000000, 0.9238795325112857393, 1.000000000000001110 ) ) 
 REPRESENTATION_ITEM ( '' )  );
#3241=CARTESIAN_POINT ( 'NONE',  ( -1.846868145590734756, -27.37500000136559564, -4.458734125000000326 ) ) ;
#3247=ORIENTED_EDGE ( 'NONE', *, *, #15306, .T. ) ;
#3274=CARTESIAN_POINT ( 'NONE',  ( -3.535533905932737309, -30.62500000000000000, -3.535533905932738197 ) ) ;
#3285=DIRECTION ( 'NONE',  ( 0.000000000000000000, 1.000000000000000000, 0.000000000000000000 ) ) ;
#3288=CARTESIAN_POINT ( 'NONE',  ( 1.846868145590736310, -29.87500000136559564, 4.458734124999997661 ) ) ;
#3295=CARTESIAN_POINT ( 'NONE',  ( -4.458734124999999437, -28.18750000136559564, -5.460374474430324690E-16 ) ) ;
#3297=CIRCLE ( 'NONE', #15434, 5.000000000000000000 ) ;
#3299=DIRECTION ( 'NONE',  ( 0.000000000000000000, 0.000000000000000000, 1.000000000000000000 ) ) ;
#3300=DIRECTION ( 'NONE',  ( 0.000000000000000000, 0.000000000000000000, 1.000000000000000000 ) ) ;
#3303=CARTESIAN_POINT ( 'NONE',  ( -3.535533905932737309, -26.62500000000000000, -3.535533905932738197 ) ) ;
#3308=DIRECTION ( 'NONE',  ( 0.000000000000000000, 0.000000000000000000, 1.000000000000000000 ) ) ;
#3309=CARTESIAN_POINT ( 'NONE',  ( 2.071067811865475505, -21.93750000273119127, -5.000000000000000888 ) ) ;
#3311=CARTESIAN_POINT ( 'NONE',  ( 1.846868145590735200, -22.25000000136559564, -4.458734124999999437 ) ) ;
#3314=CARTESIAN_POINT ( 'NONE',  ( 0.000000000000000000, 40.00000000000000000, 0.000000000000000000 ) ) ;
#3319=CARTESIAN_POINT ( 'NONE',  ( 4.458734125000000326, -29.37500000136559208, -1.846868145590734978 ) ) ;
#3320=CYLINDRICAL_SURFACE ( 'NONE', #14860, 5.000000000000000000 ) ;
#3321=EDGE_LOOP ( 'NONE', ( #11251, #11938, #8241, #4990 ) ) ;
#3324=DIRECTION ( 'NONE',  ( 0.000000000000000000, 1.000000000000000000, 0.000000000000000000 ) ) ;
#3325=CARTESIAN_POINT ( 'NONE',  ( 3.152801135295367541, -27.56250000136559564, -3.152801135295367541 ) ) ;
#3327=EDGE_CURVE ( 'NONE', #379, #2190, #12096, .T. ) ;
#3336=ORIENTED_EDGE ( 'NONE', *, *, #1140, .F. ) ;
#3339=CARTESIAN_POINT ( 'NONE',  ( 35.00000000000000000, 40.00000000000000000, -8.572527594031472993E-15 ) ) ;
#3345=CARTESIAN_POINT ( 'NONE',  ( 5.000000000000000000, -22.18750000273118772, 2.071067811865478614 ) ) ;
#3356=CARTESIAN_POINT ( 'NONE',  ( 24.26932219902320043, 20.00000000000000000, -5.999999999999989342 ) ) ;
#3365=CARTESIAN_POINT ( 'NONE',  ( 3.152801135295366208, -30.81250000136559564, 3.152801135295367985 ) ) ;
#3368=VERTEX_POINT ( 'NONE', #3431 ) ;
#3372=ORIENTED_EDGE ( 'NONE', *, *, #1820, .T. ) ;
#3373=CARTESIAN_POINT ( 'NONE',  ( 1.846868145590736310, -25.87500000136559919, 4.458734124999999437 ) ) ;
#3374=CARTESIAN_POINT ( 'NONE',  ( 0.000000000000000000, -20.00000000000000000, 0.000000000000000000 ) ) ;
#3381=CARTESIAN_POINT ( 'NONE',  ( -9.184850993605147944E-16, -21.37500000273118772, 5.000000000000000000 ) ) ;
#3384=DIRECTION ( 'NONE',  ( 0.000000000000000000, 0.000000000000000000, 1.000000000000000000 ) ) ;
#3388=PLANE ( 'NONE',  #6702 ) ;
#3389=CARTESIAN_POINT ( 'NONE',  ( 3.152801135295367541, -29.31250000136559208, -3.152801135295367541 ) ) ;
#3395=CARTESIAN_POINT ( 'NONE',  ( 2.730187237215162345E-16, -23.43750000136559564, -4.458734124999999437 ) ) ;
#3408=CARTESIAN_POINT ( 'NONE',  ( -24.26932219902320043, 20.00000000000000000, -5.999999999999984901 ) ) ;
#3419=VERTEX_POINT ( 'NONE', #13682 ) ;
#3420=VECTOR ( 'NONE', #3324, 1000.000000000000000 ) ;
#3431=CARTESIAN_POINT ( 'NONE',  ( -9.184850993605147944E-16, -30.25000000000000000, 5.000000000000000000 ) ) ;
#3432=CARTESIAN_POINT ( 'NONE',  ( -4.458734124999999437, -30.25000000136559919, -1.846868145590735644 ) ) ;
#3437=ORIENTED_EDGE ( 'NONE', *, *, #8142, .T. ) ;
#3440=CARTESIAN_POINT ( 'NONE',  ( -3.152801135295367985, -26.06250000136559919, 3.152801135295367096 ) ) ;
#3443=EDGE_CURVE ( 'NONE', #1108, #11572, #14901, .T. ) ;
#3448=CARTESIAN_POINT ( 'NONE',  ( -2.071067811865478170, -23.31249999999999645, 5.000000000000000000 ) ) ;
#3451=CARTESIAN_POINT ( 'NONE',  ( -9.184850993605147944E-16, -27.25000000000000000, 5.000000000000000000 ) ) ;
#3452=CARTESIAN_POINT ( 'NONE',  ( -8.190561711645485556E-16, -30.68750000136559564, 4.458734124999999437 ) ) ;
#3455=VERTEX_POINT ( 'NONE', #216 ) ;
#3459=CARTESIAN_POINT ( 'NONE',  ( 4.458734124999999437, -27.50000000136559208, 1.846868145590737864 ) ) ;
#3468=CARTESIAN_POINT ( 'NONE',  ( 3.152801135295367541, -23.56250000136559564, -3.152801135295367541 ) ) ;
#3482=CYLINDRICAL_SURFACE ( 'NONE', #7462, 2.649999999999992806 ) ;
#3483=CARTESIAN_POINT ( 'NONE',  ( 5.000000000000000888, -27.93750000000000711, -2.071067811865475505 ) ) ;
#3489=VERTEX_POINT ( 'NONE', #2779 ) ;
#3491=SURFACE_SIDE_STYLE ('',( #2432 ) ) ;
#3493=ORIENTED_EDGE ( 'NONE', *, *, #13493, .T. ) ;
#3496=ORIENTED_EDGE ( 'NONE', *, *, #10229, .F. ) ;
#3508=CARTESIAN_POINT ( 'NONE',  ( 2.730187237215162345E-16, -27.43750000136559564, -4.458734124999999437 ) ) ;
#3510=VERTEX_POINT ( 'NONE', #2931 ) ;
#3516=VECTOR ( 'NONE', #9867, 1000.000000000000000 ) ;
#3517=ORIENTED_EDGE ( 'NONE', *, *, #12522, .T. ) ;
#3519=CARTESIAN_POINT ( 'NONE',  ( 2.730187237215162345E-16, -23.43750000136559564, -4.458734124999999437 ) ) ;
#3520=CARTESIAN_POINT ( 'NONE',  ( 24.26932219902320043, 37.00000000000000000, -5.999999999999989342 ) ) ;
#3521=CARTESIAN_POINT ( 'NONE',  ( 3.535533905932736864, -30.25000000273118417, 3.535533905932738641 ) ) ;
#3525=CARTESIAN_POINT ( 'NONE',  ( 5.000000000000000888, -23.93750000000000000, -2.071067811865475505 ) ) ;
#3526=CARTESIAN_POINT ( 'NONE',  ( 5.000000000000000000, -23.00000000000000000, 0.000000000000000000 ) ) ;
#3530=CARTESIAN_POINT ( 'NONE',  ( 3.061616997868383141E-16, -29.75000000000000000, -5.000000000000000000 ) ) ;
#3531=CARTESIAN_POINT ( 'NONE',  ( 4.458734125000000326, -31.37500000136559564, -1.846868145590734978 ) ) ;
#3536=ORIENTED_EDGE ( 'NONE', *, *, #521, .T. ) ;
#3538=CARTESIAN_POINT ( 'NONE',  ( 35.00000000000000000, 37.00000000000000000, 5.999999999999991118 ) ) ;
#3539=CARTESIAN_POINT ( 'NONE',  ( 3.152801135295366208, -24.56250000136559564, 3.152801135295367985 ) ) ;
#3549=CARTESIAN_POINT ( 'NONE',  ( 1.846868145590736310, -21.87500000136559208, 4.458734124999999437 ) ) ;
#3552=CARTESIAN_POINT ( 'NONE',  ( -5.000000000000000000, -30.62500000273118772, -6.123233995736766282E-16 ) ) ;
#3556=EDGE_CURVE ( 'NONE', #9570, #14100, #11185, .T. ) ;
#3557=CARTESIAN_POINT ( 'NONE',  ( 5.000000000000000000, -25.00000000000000000, 0.000000000000000000 ) ) ;
#3561=( BOUNDED_CURVE ( )  B_SPLINE_CURVE ( 2, ( #962, #13450, #69, #12094, #15831, #6045, #11058, #2322, #3451 ),
 .UNSPECIFIED., .F., .F. ) 
 B_SPLINE_CURVE_WITH_KNOTS ( ( 3, 2, 2, 2, 3 ),
 ( 0.4250000000000000444, 0.4375000000000000555, 0.4500000000000000666, 0.4625000000000001332, 0.4750000000000000888 ),
 .UNSPECIFIED. ) 
 CURVE ( )  GEOMETRIC_REPRESENTATION_ITEM ( )  RATIONAL_B_SPLINE_CURVE ( ( 0.9999999999999996669, 0.9238795325112870716, 1.000000000000000000, 0.9238795325112867385, 1.000000000000000000, 0.9238795325112867385, 1.000000000000000000, 0.9238795325112860723, 1.000000000000000666 ) ) 
 REPRESENTATION_ITEM ( '' )  );
#3583=( NAMED_UNIT ( * ) SI_UNIT ( $, .STERADIAN. ) SOLID_ANGLE_UNIT ( ) );
#3584=ORIENTED_EDGE ( 'NONE', *, *, #12499, .T. ) ;
#3587=EDGE_LOOP ( 'NONE', ( #3437, #15387, #13232, #5362, #6922, #8413, #13387, #9883, #9796, #1948, #5504, #9724, #4012, #3081, #7745, #357, #8664, #12813, #11686, #776, #7888, #484, #2349, #7079 ) ) ;
#3592=CARTESIAN_POINT ( 'NONE',  ( -9.184850993605147944E-16, -29.25000000000000000, 5.000000000000000000 ) ) ;
#3593=FACE_OUTER_BOUND ( 'NONE', #1006, .T. ) ;
#3599=CARTESIAN_POINT ( 'NONE',  ( 4.458734124999999437, -24.62500000136559564, -1.846868145590734978 ) ) ;
#3600=CARTESIAN_POINT ( 'NONE',  ( -3.152801135295367096, -23.06250000136559564, -3.152801135295367541 ) ) ;
#3605=ORIENTED_EDGE ( 'NONE', *, *, #9405, .T. ) ;
#3606=CARTESIAN_POINT ( 'NONE',  ( -4.458734125000001214, -24.12500000136559919, 1.846868145590734089 ) ) ;
#3614=CARTESIAN_POINT ( 'NONE',  ( 2.071067811865476394, -23.18750000000000000, 5.000000000000000000 ) ) ;
#3617=CARTESIAN_POINT ( 'NONE',  ( -9.184850993605147944E-16, -29.25000000000000000, 5.000000000000000000 ) ) ;
#3618=CARTESIAN_POINT ( 'NONE',  ( -4.458734125000001214, -25.87500000136559919, 1.846868145590734089 ) ) ;
#3622=CARTESIAN_POINT ( 'NONE',  ( 0.000000000000000000, 40.00000000000000000, 0.000000000000000000 ) ) ;
#3626=CARTESIAN_POINT ( 'NONE',  ( -4.458734124999999437, -24.93750000136559564, -5.460374474430324690E-16 ) ) ;
#3629=DIRECTION ( 'NONE',  ( 0.000000000000000000, 1.000000000000000000, 0.000000000000000000 ) ) ;
#3635=CARTESIAN_POINT ( 'NONE',  ( 3.152801135295366208, -24.81250000136559564, 3.152801135295367985 ) ) ;
#3638=CARTESIAN_POINT ( 'NONE',  ( 5.000000000000000000, -28.12500000273118772, 0.000000000000000000 ) ) ;
#3640=CARTESIAN_POINT ( 'NONE',  ( -8.190561711645485556E-16, -30.68750000136559564, 4.458734124999999437 ) ) ;
#3644=CARTESIAN_POINT ( 'NONE',  ( 35.00000000000000000, 37.00000000000000000, -8.572527594031472993E-15 ) ) ;
#3646=CARTESIAN_POINT ( 'NONE',  ( 0.000000000000000000, -13.00000000000000178, 0.000000000000000000 ) ) ;
#3649=DIRECTION ( 'NONE',  ( -0.000000000000000000, -1.000000000000000000, -0.000000000000000000 ) ) ;
#3653=( BOUNDED_CURVE ( )  B_SPLINE_CURVE ( 2, ( #6121, #8631, #11049, #5606, #13525, #6450, #5222, #8792, #11362 ),
 .UNSPECIFIED., .F., .F. ) 
 B_SPLINE_CURVE_WITH_KNOTS ( ( 3, 2, 2, 2, 3 ),
 ( 0.3249999999999999556, 0.3374999999999999667, 0.3499999999999999778, 0.3624999999999999889, 0.3750000000000000000 ),
 .UNSPECIFIED. ) 
 CURVE ( )  GEOMETRIC_REPRESENTATION_ITEM ( )  RATIONAL_B_SPLINE_CURVE ( ( 1.000000000000000444, 0.9238795325112864054, 1.000000000000000000, 0.9238795325112867385, 1.000000000000000000, 0.9238795325112867385, 1.000000000000000000, 0.9238795325112867385, 1.000000000000000000 ) ) 
 REPRESENTATION_ITEM ( '' )  );
#3655=CARTESIAN_POINT ( 'NONE',  ( 2.071067811865476394, -24.18750000000000355, 5.000000000000000000 ) ) ;
#3660=EDGE_LOOP ( 'NONE', ( #15209, #2647, #3517, #8627, #809, #7575, #13814 ) ) ;
#3663=CARTESIAN_POINT ( 'NONE',  ( 6.123233995736766282E-16, -20.00000000000000000, -5.000000000000000000 ) ) ;
#3668=CARTESIAN_POINT ( 'NONE',  ( -9.184850993605147944E-16, -26.37500000273118417, 5.000000000000000000 ) ) ;
#3669=CARTESIAN_POINT ( 'NONE',  ( 0.000000000000000000, -20.00000000000000000, 0.000000000000000000 ) ) ;
#3672=CARTESIAN_POINT ( 'NONE',  ( -4.458734124999999437, -25.18750000136559564, -5.460374474430324690E-16 ) ) ;
#3677=ORIENTED_EDGE ( 'NONE', *, *, #7275, .F. ) ;
#3681=CARTESIAN_POINT ( 'NONE',  ( 4.458734124999999437, -22.68750000136559564, 0.000000000000000000 ) ) ;
#3683=CARTESIAN_POINT ( 'NONE',  ( 5.000000000000000000, -30.18750000273118417, 2.071067811865478614 ) ) ;
#3692=CARTESIAN_POINT ( 'NONE',  ( 4.458734124999999437, -25.50000000136559919, 1.846868145590737864 ) ) ;
#3700=CARTESIAN_POINT ( 'NONE',  ( -1.846868145590737420, -26.75000000136559564, 4.458734124999999437 ) ) ;
#3701=EDGE_CURVE ( 'NONE', #3157, #4598, #8127, .T. ) ;
#3708=CARTESIAN_POINT ( 'NONE',  ( 3.152801135295367541, -25.56250000136559564, -3.152801135295367541 ) ) ;
#3711=CARTESIAN_POINT ( 'NONE',  ( 2.071067811865475505, -27.93750000273119127, -5.000000000000000888 ) ) ;
#3714=CARTESIAN_POINT ( 'NONE',  ( 4.458734124999999437, -30.37500000136559564, -1.846868145590734978 ) ) ;
#3722=EDGE_CURVE ( 'NONE', #2036, #5406, #9562, .T. ) ;
#3729=CARTESIAN_POINT ( 'NONE',  ( 0.000000000000000000, -20.00000000000000000, 0.000000000000000000 ) ) ;
#3750=CARTESIAN_POINT ( 'NONE',  ( -4.458734125000000326, -25.12500000136559564, 1.846868145590734089 ) ) ;
#3754=DIRECTION ( 'NONE',  ( 1.000000000000000000, -0.000000000000000000, -1.239088197126290570E-16 ) ) ;
#3758=ADVANCED_FACE ( 'NONE', ( #15869 ), #4791, .T. ) ;
#3763=CARTESIAN_POINT ( 'NONE',  ( 3.152801135295366208, -22.81250000136559564, 3.152801135295367985 ) ) ;
#3764=LINE ( 'NONE', #7500, #9971 ) ;
#3767=CARTESIAN_POINT ( 'NONE',  ( -9.184850993605147944E-16, -26.25000000000000355, 5.000000000000000000 ) ) ;
#3768=DIRECTION ( 'NONE',  ( 0.000000000000000000, 0.000000000000000000, 1.000000000000000000 ) ) ;
#3774=CARTESIAN_POINT ( 'NONE',  ( 4.458734125000000326, -28.37500000136559564, -1.846868145590734978 ) ) ;
#3777=ORIENTED_EDGE ( 'NONE', *, *, #1820, .F. ) ;
#3784=CARTESIAN_POINT ( 'NONE',  ( -1.846868145590737420, -25.75000000136559564, 4.458734124999999437 ) ) ;
#3792=CARTESIAN_POINT ( 'NONE',  ( 0.000000000000000000, -13.00000000000000178, 0.000000000000000000 ) ) ;
#3793=CARTESIAN_POINT ( 'NONE',  ( -5.000000000000000000, -28.50000000000000000, -6.123233995736766282E-16 ) ) ;
#3798=CARTESIAN_POINT ( 'NONE',  ( -2.071067811865475061, -26.81250000273118417, -5.000000000000000888 ) ) ;
#3800=CARTESIAN_POINT ( 'NONE',  ( 3.535533905932738197, -24.00000000273118772, -3.535533905932738197 ) ) ;
#3806=CARTESIAN_POINT ( 'NONE',  ( -35.00000000000000000, 37.00000000000000000, -2.649999999999992806 ) ) ;
#3816=CIRCLE ( 'NONE', #10021, 6.000000000000000888 ) ;
#3822=ORIENTED_EDGE ( 'NONE', *, *, #12125, .F. ) ;
#3830=LINE ( 'NONE', #14742, #9275 ) ;
#3839=CARTESIAN_POINT ( 'NONE',  ( -3.152801135295367985, -26.06250000136559919, 3.152801135295367096 ) ) ;
#3840=ORIENTED_EDGE ( 'NONE', *, *, #8774, .F. ) ;
#3847=AXIS2_PLACEMENT_3D ( 'NONE', #5001, #8735, #1442 ) ;
#3849=CARTESIAN_POINT ( 'NONE',  ( 1.846868145590735200, -23.50000000136559564, -4.458734125000000326 ) ) ;
#3850=DIRECTION ( 'NONE',  ( 0.000000000000000000, 0.000000000000000000, 1.000000000000000000 ) ) ;
#3852=CARTESIAN_POINT ( 'NONE',  ( 0.000000000000000000, -13.00000000000000178, 0.000000000000000000 ) ) ;
#3854=CARTESIAN_POINT ( 'NONE',  ( 2.071067811865462183, -26.18750000000000711, 5.000000000000013323 ) ) ;
#3856=ADVANCED_FACE ( 'NONE', ( #12448 ), #11484, .F. ) ;
#3859=CARTESIAN_POINT ( 'NONE',  ( 0.000000000000000000, -20.00000000000000000, 0.000000000000000000 ) ) ;
#3861=CARTESIAN_POINT ( 'NONE',  ( -4.458734124999999437, -24.93750000136559564, -5.460374474430324690E-16 ) ) ;
#3865=ORIENTED_EDGE ( 'NONE', *, *, #7478, .F. ) ;
#3867=DIRECTION ( 'NONE',  ( -0.000000000000000000, 1.000000000000000000, -0.000000000000000000 ) ) ;
#3868=CARTESIAN_POINT ( 'NONE',  ( -8.190561711645485556E-16, -24.68750000136559564, 4.458734124999999437 ) ) ;
#3873=CYLINDRICAL_SURFACE ( 'NONE', #3847, 5.000000000000000000 ) ;
#3877=CARTESIAN_POINT ( 'NONE',  ( 3.061616997868383141E-16, -29.75000000000000000, -5.000000000000000000 ) ) ;
#3880=CARTESIAN_POINT ( 'NONE',  ( -3.535533905932738641, -26.50000000273118772, 3.535533905932737309 ) ) ;
#3882=CARTESIAN_POINT ( 'NONE',  ( -4.458734124999999437, -29.93750000136559564, -5.460374474430324690E-16 ) ) ;
#3887=ORIENTED_EDGE ( 'NONE', *, *, #8774, .T. ) ;
#3889=FACE_OUTER_BOUND ( 'NONE', #3587, .T. ) ;
#3895=FACE_OUTER_BOUND ( 'NONE', #6640, .T. ) ;
#3905=CARTESIAN_POINT ( 'NONE',  ( -5.000000000000000888, -28.68750000273119127, -2.071067811865475949 ) ) ;
#3906=DIRECTION ( 'NONE',  ( 0.000000000000000000, 0.000000000000000000, 1.000000000000000000 ) ) ;
#3912=CARTESIAN_POINT ( 'NONE',  ( 4.458734124999999437, -22.62500000136559564, -1.846868145590734978 ) ) ;
#3914=DIRECTION ( 'NONE',  ( -0.000000000000000000, -1.000000000000000000, -0.000000000000000000 ) ) ;
#3917=ORIENTED_EDGE ( 'NONE', *, *, #7796, .F. ) ;
#3919=CIRCLE ( 'NONE', #8071, 5.000000000000000000 ) ;
#3921=CYLINDRICAL_SURFACE ( 'NONE', #8223, 5.000000000000000000 ) ;
#3933=CARTESIAN_POINT ( 'NONE',  ( -3.152801135295367985, -23.81250000136559564, 3.152801135295367096 ) ) ;
#3939=CARTESIAN_POINT ( 'NONE',  ( 3.152801135295367541, -29.56250000136559208, -3.152801135295367541 ) ) ;
#3940=EDGE_CURVE ( 'NONE', #15165, #4719, #8920, .T. ) ;
#3950=CARTESIAN_POINT ( 'NONE',  ( 3.535533905932738197, -29.87500000000000000, -3.535533905932738197 ) ) ;
#3954=CARTESIAN_POINT ( 'NONE',  ( -2.071067811865478170, -29.43750000273118772, 5.000000000000000000 ) ) ;
#3966=CARTESIAN_POINT ( 'NONE',  ( -1.846868145590737420, -30.00000000136559564, 4.458734124999999437 ) ) ;
#3980=LINE ( 'NONE', #3408, #251 ) ;
#3988=LINE ( 'NONE', #10070, #13013 ) ;
#3993=VERTEX_POINT ( 'NONE', #14319 ) ;
#3994=ORIENTED_EDGE ( 'NONE', *, *, #9740, .F. ) ;
#4002=CARTESIAN_POINT ( 'NONE',  ( 5.000000000000000000, -26.00000000000000355, 0.000000000000000000 ) ) ;
#4010=CARTESIAN_POINT ( 'NONE',  ( -4.458734124999999437, -22.93750000136559564, -5.460374474430324690E-16 ) ) ;
#4012=ORIENTED_EDGE ( 'NONE', *, *, #14328, .T. ) ;
#4014=VERTEX_POINT ( 'NONE', #3003 ) ;
#4018=CARTESIAN_POINT ( 'NONE',  ( -8.190561711645485556E-16, -22.68750000136559564, 4.458734124999999437 ) ) ;
#4027=CARTESIAN_POINT ( 'NONE',  ( 3.535533905932738197, -28.87500000000000000, -3.535533905932738197 ) ) ;
#4032=CARTESIAN_POINT ( 'NONE',  ( 3.061616997868383141E-16, -22.87500000273118772, -5.000000000000000000 ) ) ;
#4034=CARTESIAN_POINT ( 'NONE',  ( 1.846868145590735200, -27.25000000136559564, -4.458734124999999437 ) ) ;
#4081=( BOUNDED_CURVE ( )  B_SPLINE_CURVE ( 2, ( #12308, #14918, #7568, #50, #9979, #12465, #2695, #12630, #217 ),
 .UNSPECIFIED., .F., .F. ) 
 B_SPLINE_CURVE_WITH_KNOTS ( ( 3, 2, 2, 2, 3 ),
 ( 0.2749999999999999112, 0.2874999999999998668, 0.2999999999999999334, 0.3124999999999999445, 0.3249999999999999556 ),
 .UNSPECIFIED. ) 
 CURVE ( )  GEOMETRIC_REPRESENTATION_ITEM ( )  RATIONAL_B_SPLINE_CURVE ( ( 1.000000000000000666, 0.9238795325112860723, 1.000000000000000000, 0.9238795325112867385, 1.000000000000000000, 0.9238795325112867385, 1.000000000000000000, 0.9238795325112870716, 0.9999999999999996669 ) ) 
 REPRESENTATION_ITEM ( '' )  );
#4089=CARTESIAN_POINT ( 'NONE',  ( 35.00000000000000000, 37.00000000000000000, 5.999999999999991118 ) ) ;
#4090=DIRECTION ( 'NONE',  ( 0.000000000000000000, 0.000000000000000000, -1.000000000000000000 ) ) ;
#4094=CIRCLE ( 'NONE', #6171, 5.999999999999991118 ) ;
#4100=CARTESIAN_POINT ( 'NONE',  ( 0.000000000000000000, -11.00000000000000178, 0.000000000000000000 ) ) ;
#4102=ORIENTED_EDGE ( 'NONE', *, *, #6738, .F. ) ;
#4104=CARTESIAN_POINT ( 'NONE',  ( 1.846868145590736310, -29.87500000136559564, 4.458734124999999437 ) ) ;
#4113=DIRECTION ( 'NONE',  ( 0.000000000000000000, 0.000000000000000000, 1.000000000000000000 ) ) ;
#4114=CARTESIAN_POINT ( 'NONE',  ( 2.071067811865476394, -31.18750000000000355, 5.000000000000000000 ) ) ;
#4117=CARTESIAN_POINT ( 'NONE',  ( 3.061616997868383141E-16, -26.75000000000000000, -5.000000000000000000 ) ) ;
#4118=CARTESIAN_POINT ( 'NONE',  ( -3.535533905932738641, -22.50000000273118772, 3.535533905932737309 ) ) ;
#4120=CARTESIAN_POINT ( 'NONE',  ( 4.458734124999999437, -27.37500000136559564, -1.846868145590734978 ) ) ;
#4127=FACE_OUTER_BOUND ( 'NONE', #6244, .T. ) ;
#4132=CARTESIAN_POINT ( 'NONE',  ( 4.458734124999999437, -31.68750000136559564, 0.000000000000000000 ) ) ;
#4136=VERTEX_POINT ( 'NONE', #14422 ) ;
#4150=CARTESIAN_POINT ( 'NONE',  ( -5.000000000000000888, -23.43749999999999645, 2.071067811865474617 ) ) ;
#4152=CARTESIAN_POINT ( 'NONE',  ( 3.152801135295367541, -22.56250000136559564, -3.152801135295367541 ) ) ;
#4166=CARTESIAN_POINT ( 'NONE',  ( -9.184850993605147944E-16, -26.37500000273118417, 5.000000000000000000 ) ) ;
#4173=CARTESIAN_POINT ( 'NONE',  ( 5.000000000000000000, -25.12500000273118417, 0.000000000000000000 ) ) ;
#4174=CARTESIAN_POINT ( 'NONE',  ( -4.458734125000000326, -23.00000000136559564, -1.846868145590735644 ) ) ;
#4183=CARTESIAN_POINT ( 'NONE',  ( 4.458734125000000326, -31.62500000136559564, -1.846868145590734978 ) ) ;
#4189=CARTESIAN_POINT ( 'NONE',  ( 4.458734124999999437, -21.68750000136559208, 0.000000000000000000 ) ) ;
#4191=CARTESIAN_POINT ( 'NONE',  ( -2.071067811865475061, -25.68750000000000355, -5.000000000000000888 ) ) ;
#4194=CARTESIAN_POINT ( 'NONE',  ( 35.00000000000000000, 37.00000000000000000, 2.649999999999983924 ) ) ;
#4195=CARTESIAN_POINT ( 'NONE',  ( 5.000000000000000000, -23.12500000273118772, 0.000000000000000000 ) ) ;
#4197=CARTESIAN_POINT ( 'NONE',  ( -4.458734124999999437, -25.93750000136559564, -5.460374474430324690E-16 ) ) ;
#4204=CIRCLE ( 'NONE', #2907, 5.000000000000000000 ) ;
#4207=DIRECTION ( 'NONE',  ( -0.000000000000000000, 1.000000000000000000, -0.000000000000000000 ) ) ;
#4208=PRODUCT ( 'Drive Unit', 'Drive Unit', '', ( #11715 ) ) ;
#4210=CARTESIAN_POINT ( 'NONE',  ( -3.152801135295367985, -28.06250000136559564, 3.152801135295367096 ) ) ;
#4221=CARTESIAN_POINT ( 'NONE',  ( 3.152801135295367541, -28.31250000136559564, -3.152801135295367541 ) ) ;
#4224=AXIS2_PLACEMENT_3D ( 'NONE', #8780, #9025, #4229 ) ;
#4226=CARTESIAN_POINT ( 'NONE',  ( 0.000000000000000000, -13.00000000000000178, 0.000000000000000000 ) ) ;
#4229=DIRECTION ( 'NONE',  ( 0.000000000000000000, 0.000000000000000000, 1.000000000000000000 ) ) ;
#4232=DIRECTION ( 'NONE',  ( -0.000000000000000000, 1.000000000000000000, -0.000000000000000000 ) ) ;
#4237=DIRECTION ( 'NONE',  ( -0.000000000000000000, 1.000000000000000000, -0.000000000000000000 ) ) ;
#4250=CARTESIAN_POINT ( 'NONE',  ( 3.061616997868383141E-16, -22.75000000000000000, -5.000000000000000000 ) ) ;
#4251=LINE ( 'NONE', #9198, #7166 ) ;
#4252=LINE ( 'NONE', #1825, #8364 ) ;
#4256=CARTESIAN_POINT ( 'NONE',  ( -1.846868145590737420, -22.75000000136559208, 4.458734124999999437 ) ) ;
#4261=ORIENTED_EDGE ( 'NONE', *, *, #8019, .T. ) ;
#4266=CARTESIAN_POINT ( 'NONE',  ( -8.190561711645485556E-16, -29.93750000136559564, 4.458734124999999437 ) ) ;
#4270=DIRECTION ( 'NONE',  ( 0.000000000000000000, 1.000000000000000000, 0.000000000000000000 ) ) ;
#4275=CARTESIAN_POINT ( 'NONE',  ( 5.000000000000000000, -25.06250000000000355, 2.071067811865478614 ) ) ;
#4280=CARTESIAN_POINT ( 'NONE',  ( -5.000000000000000888, -25.56250000273118417, 2.071067811865474617 ) ) ;
#4284=VECTOR ( 'NONE', #4270, 1000.000000000000000 ) ;
#4285=CARTESIAN_POINT ( 'NONE',  ( 4.458734124999997661, -26.50000000136559564, 1.846868145590737864 ) ) ;
#4291=CARTESIAN_POINT ( 'NONE',  ( 3.535533905932738197, -29.00000000273118772, -3.535533905932738197 ) ) ;
#4297=CARTESIAN_POINT ( 'NONE',  ( 3.061616997868383141E-16, -31.75000000000000000, -5.000000000000000000 ) ) ;
#4298=CARTESIAN_POINT ( 'NONE',  ( -8.190561711645485556E-16, -27.93750000136559564, 4.458734124999999437 ) ) ;
#4309=VECTOR ( 'NONE', #13445, 1000.000000000000000 ) ;
#4314=DIRECTION ( 'NONE',  ( 1.000000000000000000, 0.000000000000000000, 0.000000000000000000 ) ) ;
#4334=FACE_BOUND ( 'NONE', #8727, .T. ) ;
#4339=CARTESIAN_POINT ( 'NONE',  ( 2.071067811865491048, -26.31250000273118417, 4.999999999999985789 ) ) ;
#4343=CARTESIAN_POINT ( 'NONE',  ( 3.061616997868383141E-16, -27.75000000000000000, -5.000000000000000000 ) ) ;
#4345=CARTESIAN_POINT ( 'NONE',  ( 1.846868145590736310, -28.87500000136559564, 4.458734124999997661 ) ) ;
#4352=CARTESIAN_POINT ( 'NONE',  ( -1.846868145590734756, -25.37500000136559919, -4.458734125000000326 ) ) ;
#4355=AXIS2_PLACEMENT_3D ( 'NONE', #4226, #9168, #3016 ) ;
#4356=CARTESIAN_POINT ( 'NONE',  ( 0.000000000000000000, -20.00000000000000000, 0.000000000000000000 ) ) ;
#4365=CARTESIAN_POINT ( 'NONE',  ( 5.000000000000000000, -26.06250000000000355, 2.071067811865478614 ) ) ;
#4369=CARTESIAN_POINT ( 'NONE',  ( 2.071067811865475505, -24.93750000273118772, -5.000000000000000888 ) ) ;
#4372=CARTESIAN_POINT ( 'NONE',  ( -4.458734124999999437, -27.93750000136559564, -5.460374474430324690E-16 ) ) ;
#4378=AXIS2_PLACEMENT_3D ( 'NONE', #3538, #8494, #2329 ) ;
#4383=CARTESIAN_POINT ( 'NONE',  ( 4.458734124999999437, -25.75000000136559564, 1.846868145590737864 ) ) ;
#4387=CARTESIAN_POINT ( 'NONE',  ( 2.071067811865473285, -31.81249999999999289, -5.000000000000002665 ) ) ;
#4390=EDGE_LOOP ( 'NONE', ( #12843, #346, #15608, #8435 ) ) ;
#4394=ORIENTED_EDGE ( 'NONE', *, *, #13923, .T. ) ;
#4401=SURFACE_STYLE_FILL_AREA ( #2855 ) ;
#4406=ADVANCED_FACE ( 'NONE', ( #14764 ), #9831, .T. ) ;
#4407=ORIENTED_EDGE ( 'NONE', *, *, #8541, .F. ) ;
#4411=CARTESIAN_POINT ( 'NONE',  ( -9.184850993605147944E-16, -23.37500000273118772, 5.000000000000000000 ) ) ;
#4416=CARTESIAN_POINT ( 'NONE',  ( 2.071067811865447528, -22.81250000000000000, -5.000000000000029310 ) ) ;
#4418=DIRECTION ( 'NONE',  ( -0.000000000000000000, 1.000000000000000000, -0.000000000000000000 ) ) ;
#4420=CARTESIAN_POINT ( 'NONE',  ( -4.458734124999999437, -29.25000000136559564, -1.846868145590735644 ) ) ;
#4427=EDGE_CURVE ( 'NONE', #2056, #4537, #1264, .T. ) ;
#4429=CARTESIAN_POINT ( 'NONE',  ( 4.458734125000000326, -27.62500000136559564, -1.846868145590734978 ) ) ;
#4435=CARTESIAN_POINT ( 'NONE',  ( -5.000000000000000000, -25.50000000000000355, -6.123233995736766282E-16 ) ) ;
#4439=CARTESIAN_POINT ( 'NONE',  ( 3.152801135295366208, -29.56250000136559208, 3.152801135295367985 ) ) ;
#4441=CARTESIAN_POINT ( 'NONE',  ( 4.458734124999999437, -21.43750000136559208, 0.000000000000000000 ) ) ;
#4445=ORIENTED_EDGE ( 'NONE', *, *, #15324, .T. ) ;
#4447=EDGE_CURVE ( 'NONE', #5406, #13669, #1583, .T. ) ;
#4453=CARTESIAN_POINT ( 'NONE',  ( -1.846868145590734756, -28.37500000136559564, -4.458734125000000326 ) ) ;
#4463=ORIENTED_EDGE ( 'NONE', *, *, #8142, .F. ) ;
#4483=ORIENTED_EDGE ( 'NONE', *, *, #8975, .F. ) ;
#4484=ORIENTED_EDGE ( 'NONE', *, *, #6938, .T. ) ;
#4485=CARTESIAN_POINT ( 'NONE',  ( -5.000000000000000888, -30.56250000000000000, -2.071067811865475949 ) ) ;
#4496=CARTESIAN_POINT ( 'NONE',  ( -3.152801135295367985, -31.06250000136559564, 3.152801135295367096 ) ) ;
#4502=CARTESIAN_POINT ( 'NONE',  ( 3.152801135295366208, -26.81250000136559564, 3.152801135295367985 ) ) ;
#4506=CARTESIAN_POINT ( 'NONE',  ( -5.000000000000000888, -29.43750000000000711, 2.071067811865474617 ) ) ;
#4507=EDGE_CURVE ( 'NONE', #12690, #3419, #5064, .T. ) ;
#4511=CARTESIAN_POINT ( 'NONE',  ( 5.000000000000000000, -27.06250000000000000, 2.071067811865478614 ) ) ;
#4515=CARTESIAN_POINT ( 'NONE',  ( -3.152801135295367985, -30.81250000136559564, 3.152801135295367096 ) ) ;
#4518=CARTESIAN_POINT ( 'NONE',  ( 1.846868145590736310, -23.62500000136559564, 4.458734124999997661 ) ) ;
#4522=VECTOR ( 'NONE', #5281, 1000.000000000000000 ) ;
#4524=CARTESIAN_POINT ( 'NONE',  ( 4.458734124999999437, -28.50000000136559564, 1.846868145590737864 ) ) ;
#4532=CARTESIAN_POINT ( 'NONE',  ( -3.152801135295367096, -28.31250000136559564, -3.152801135295367541 ) ) ;
#4533=DIRECTION ( 'NONE',  ( 0.000000000000000000, 0.000000000000000000, -1.000000000000000000 ) ) ;
#4534=DIRECTION ( 'NONE',  ( -0.000000000000000000, 1.000000000000000000, -0.000000000000000000 ) ) ;
#4537=VERTEX_POINT ( 'NONE', #4089 ) ;
#4543=CARTESIAN_POINT ( 'NONE',  ( -5.000000000000000888, -26.56250000000000000, -2.071067811865475949 ) ) ;
#4574=CARTESIAN_POINT ( 'NONE',  ( -8.190561711645485556E-16, -28.93750000136559564, 4.458734124999999437 ) ) ;
#4581=CARTESIAN_POINT ( 'NONE',  ( -1.846868145590734756, -28.37500000136559564, -4.458734125000000326 ) ) ;
#4593=CARTESIAN_POINT ( 'NONE',  ( -3.152801135295367985, -28.81250000136559564, 3.152801135295367096 ) ) ;
#4598=VERTEX_POINT ( 'NONE', #1744 ) ;
#4601=CARTESIAN_POINT ( 'NONE',  ( 3.152801135295366208, -30.56250000136559564, 3.152801135295367985 ) ) ;
#4603=DIRECTION ( 'NONE',  ( -0.000000000000000000, 1.000000000000000000, -0.000000000000000000 ) ) ;
#4604=( BOUNDED_CURVE ( )  B_SPLINE_CURVE ( 2, ( #13273, #2302, #13199, #1162, #15809, #2065, #6104, #12147, #2214 ),
 .UNSPECIFIED., .F., .F. ) 
 B_SPLINE_CURVE_WITH_KNOTS ( ( 3, 2, 2, 2, 3 ),
 ( 0.1250000000000001110, 0.1375000000000001221, 0.1500000000000001332, 0.1625000000000001443, 0.1750000000000001554 ),
 .UNSPECIFIED. ) 
 CURVE ( )  GEOMETRIC_REPRESENTATION_ITEM ( )  RATIONAL_B_SPLINE_CURVE ( ( 0.9999999999999993339, 0.9238795325112874046, 1.000000000000000000, 0.9238795325112867385, 1.000000000000000000, 0.9238795325112867385, 1.000000000000000000, 0.9238795325112857393, 1.000000000000001110 ) ) 
 REPRESENTATION_ITEM ( '' )  );
#4613=CARTESIAN_POINT ( 'NONE',  ( 1.846868145590736310, -23.87500000136559564, 4.458734124999999437 ) ) ;
#4615=CYLINDRICAL_SURFACE ( 'NONE', #6248, 25.00000000000000000 ) ;
#4620=VERTEX_POINT ( 'NONE', #14113 ) ;
#4626=ADVANCED_FACE ( 'NONE', ( #1981 ), #14353, .T. ) ;
#4628=CARTESIAN_POINT ( 'NONE',  ( -9.184850993605147944E-16, -26.25000000000000355, 5.000000000000000000 ) ) ;
#4638=DIRECTION ( 'NONE',  ( 1.000000000000000000, 0.000000000000000000, 0.000000000000000000 ) ) ;
#4647=CARTESIAN_POINT ( 'NONE',  ( 0.000000000000000000, 40.00000000000000000, 0.000000000000000000 ) ) ;
#4649=CARTESIAN_POINT ( 'NONE',  ( -9.184850993605147944E-16, -25.25000000000000000, 5.000000000000000000 ) ) ;
#4652=CARTESIAN_POINT ( 'NONE',  ( -2.071067811865475061, -24.68750000000000355, -5.000000000000000888 ) ) ;
#4653=CARTESIAN_POINT ( 'NONE',  ( -3.535533905932738641, -22.50000000273118772, 3.535533905932737309 ) ) ;
#4654=CARTESIAN_POINT ( 'NONE',  ( 4.458734124999999437, -30.68750000136559564, 0.000000000000000000 ) ) ;
#4663=VERTEX_POINT ( 'NONE', #5628 ) ;
#4664=CARTESIAN_POINT ( 'NONE',  ( -1.846868145590734756, -27.37500000136559564, -4.458734125000000326 ) ) ;
#4668=CARTESIAN_POINT ( 'NONE',  ( 0.000000000000000000, -13.00000000000000178, 1.500000000000000000 ) ) ;
#4669=CARTESIAN_POINT ( 'NONE',  ( -3.535533905932738641, -23.37500000000000000, 3.535533905932737309 ) ) ;
#4673=CARTESIAN_POINT ( 'NONE',  ( 3.152801135295367541, -31.31250000136559564, -3.152801135295367541 ) ) ;
#4678=FACE_OUTER_BOUND ( 'NONE', #8219, .T. ) ;
#4680=CARTESIAN_POINT ( 'NONE',  ( 4.458734124999999437, -28.43750000136559564, 0.000000000000000000 ) ) ;
#4686=LINE ( 'NONE', #1940, #3420 ) ;
#4687=CARTESIAN_POINT ( 'NONE',  ( -4.458734125000001214, -23.12500000136559564, 1.846868145590734089 ) ) ;
#4689=EDGE_CURVE ( 'NONE', #2036, #13476, #9931, .T. ) ;
#4695=( BOUNDED_CURVE ( )  B_SPLINE_CURVE ( 2, ( #8150, #14358, #11604, #8072, #4173, #555, #12893, #7907, #787 ),
 .UNSPECIFIED., .F., .F. ) 
 B_SPLINE_CURVE_WITH_KNOTS ( ( 3, 2, 2, 2, 3 ),
 ( 0.5750000000000001776, 0.5875000000000002442, 0.6000000000000001998, 0.6125000000000002665, 0.6250000000000002220 ),
 .UNSPECIFIED. ) 
 CURVE ( )  GEOMETRIC_REPRESENTATION_ITEM ( )  RATIONAL_B_SPLINE_CURVE ( ( 0.9999999999999986677, 0.9238795325112880708, 1.000000000000000000, 0.9238795325112867385, 1.000000000000000000, 0.9238795325112867385, 1.000000000000000000, 0.9238795325112854062, 1.000000000000001332 ) ) 
 REPRESENTATION_ITEM ( '' )  );
#4711=CARTESIAN_POINT ( 'NONE',  ( 3.535533905932736864, -22.25000000273118417, 3.535533905932738641 ) ) ;
#4719=VERTEX_POINT ( 'NONE', #11834 ) ;
#4722=CARTESIAN_POINT ( 'NONE',  ( 0.000000000000000000, -13.00000000000000178, -1.500000000000000000 ) ) ;
#4728=CARTESIAN_POINT ( 'NONE',  ( -3.535533905932738641, -24.37500000000000000, 3.535533905932737309 ) ) ;
#4729=CARTESIAN_POINT ( 'NONE',  ( -5.000000000000000000, -22.62500000273118772, -6.123233995736766282E-16 ) ) ;
#4730=CARTESIAN_POINT ( 'NONE',  ( 1.846868145590735200, -24.50000000136559564, -4.458734124999999437 ) ) ;
#4739=VECTOR ( 'NONE', #13046, 1000.000000000000000 ) ;
#4740=CARTESIAN_POINT ( 'NONE',  ( -4.458734124999999437, -22.18750000136559564, -5.460374474430324690E-16 ) ) ;
#4741=DIRECTION ( 'NONE',  ( -0.000000000000000000, -1.000000000000000000, -0.000000000000000000 ) ) ;
#4743=ADVANCED_FACE ( 'NONE', ( #3593 ), #10796, .T. ) ;
#4752=CARTESIAN_POINT ( 'NONE',  ( -1.846868145590734756, -30.12500000136559208, -4.458734125000000326 ) ) ;
#4759=CARTESIAN_POINT ( 'NONE',  ( -4.458734125000001214, -26.87500000136559208, 1.846868145590734089 ) ) ;
#4760=DIRECTION ( 'NONE',  ( -0.000000000000000000, 1.000000000000000000, -0.000000000000000000 ) ) ;
#4764=DIRECTION ( 'NONE',  ( 0.000000000000000000, 0.000000000000000000, -1.000000000000000000 ) ) ;
#4768=CARTESIAN_POINT ( 'NONE',  ( -3.152801135295367985, -22.06250000136559564, 3.152801135295367096 ) ) ;
#4788=( BOUNDED_CURVE ( )  B_SPLINE_CURVE ( 2, ( #11496, #14992, #445, #3905, #10311, #6430, #15238, #2774, #291 ),
 .UNSPECIFIED., .F., .F. ) 
 B_SPLINE_CURVE_WITH_KNOTS ( ( 3, 2, 2, 2, 3 ),
 ( 0.2249999999999998668, 0.2374999999999998501, 0.2499999999999998890, 0.2624999999999999001, 0.2749999999999999112 ),
 .UNSPECIFIED. ) 
 CURVE ( )  GEOMETRIC_REPRESENTATION_ITEM ( )  RATIONAL_B_SPLINE_CURVE ( ( 1.000000000000000888, 0.9238795325112858503, 1.000000000000000000, 0.9238795325112867385, 1.000000000000000000, 0.9238795325112867385, 1.000000000000000000, 0.9238795325112874046, 0.9999999999999993339 ) ) 
 REPRESENTATION_ITEM ( '' )  );
#4791=PLANE ( 'NONE',  #14105 ) ;
#4804=CARTESIAN_POINT ( 'NONE',  ( 0.000000000000000000, -11.00000000000000178, 0.000000000000000000 ) ) ;
#4806=CARTESIAN_POINT ( 'NONE',  ( -35.00000000000000000, 40.00000000000000000, 0.000000000000000000 ) ) ;
#4809=FACE_OUTER_BOUND ( 'NONE', #15645, .T. ) ;
#4814=CARTESIAN_POINT ( 'NONE',  ( -3.152801135295367096, -27.31250000136559564, -3.152801135295367541 ) ) ;
#4819=ORIENTED_EDGE ( 'NONE', *, *, #3722, .T. ) ;
#4820=CARTESIAN_POINT ( 'NONE',  ( -4.458734125000000326, -22.25000000136559564, -1.846868145590735644 ) ) ;
#4834=CARTESIAN_POINT ( 'NONE',  ( -4.458734125000001214, -27.87500000136559564, 1.846868145590734089 ) ) ;
#4837=CARTESIAN_POINT ( 'NONE',  ( 35.00000000000000000, 37.00000000000000000, 2.649999999999976819 ) ) ;
#4840=ORIENTED_EDGE ( 'NONE', *, *, #13923, .F. ) ;
#4841=FACE_OUTER_BOUND ( 'NONE', #13689, .T. ) ;
#4843=CARTESIAN_POINT ( 'NONE',  ( -3.152801135295367096, -25.06250000136559564, -3.152801135295367541 ) ) ;
#4846=EDGE_CURVE ( 'NONE', #15819, #9634, #856, .T. ) ;
#4849=FACE_BOUND ( 'NONE', #7910, .T. ) ;
#4851=VECTOR ( 'NONE', #15912, 1000.000000000000000 ) ;
#4854=CARTESIAN_POINT ( 'NONE',  ( 1.846868145590735200, -22.50000000136559208, -4.458734125000000326 ) ) ;
#4857=CARTESIAN_POINT ( 'NONE',  ( -9.184850993605147944E-16, -29.37500000273118417, 5.000000000000000000 ) ) ;
#4872=CARTESIAN_POINT ( 'NONE',  ( -3.535533905932738641, -25.50000000273118417, 3.535533905932737309 ) ) ;
#4887=( BOUNDED_CURVE ( )  B_SPLINE_CURVE ( 2, ( #4297, #8915, #13819, #2754, #351, #14162, #7863, #7711, #7621 ),
 .UNSPECIFIED., .F., .F. ) 
 B_SPLINE_CURVE_WITH_KNOTS ( ( 3, 2, 2, 2, 3 ),
 ( 0.02500000000000002220, 0.03750000000000003331, 0.05000000000000004441, 0.06250000000000005551, 0.07500000000000006661 ),
 .UNSPECIFIED. ) 
 CURVE ( )  GEOMETRIC_REPRESENTATION_ITEM ( )  RATIONAL_B_SPLINE_CURVE ( ( 0.9999999999999998890, 0.9238795325112868495, 1.000000000000000000, 0.9238795325112867385, 1.000000000000000000, 0.9238795325112867385, 1.000000000000000000, 0.9238795325112862944, 1.000000000000000444 ) ) 
 REPRESENTATION_ITEM ( '' )  );
#4895=CARTESIAN_POINT ( 'NONE',  ( 4.458734124999999437, -26.68750000136559564, 0.000000000000000000 ) ) ;
#4896=CARTESIAN_POINT ( 'NONE',  ( -1.846868145590734756, -22.12500000136559564, -4.458734124999999437 ) ) ;
#4899=ORIENTED_EDGE ( 'NONE', *, *, #5361, .F. ) ;
#4903=CARTESIAN_POINT ( 'NONE',  ( -8.190561711645485556E-16, -24.93750000136559564, 4.458734124999999437 ) ) ;
#4904=FACE_OUTER_BOUND ( 'NONE', #6076, .T. ) ;
#4913=CARTESIAN_POINT ( 'NONE',  ( -4.458734124999999437, -25.93750000136559564, -5.460374474430324690E-16 ) ) ;
#4920=CARTESIAN_POINT ( 'NONE',  ( 3.152801135295367541, -23.31250000136559564, -3.152801135295367541 ) ) ;
#4925=DIRECTION ( 'NONE',  ( 0.000000000000000000, 0.000000000000000000, 1.000000000000000000 ) ) ;
#4928=CARTESIAN_POINT ( 'NONE',  ( -1.846868145590734756, -25.37500000136559919, -4.458734125000000326 ) ) ;
#4933=CARTESIAN_POINT ( 'NONE',  ( -2.071067811865478170, -28.43750000273119127, 5.000000000000000000 ) ) ;
#4935=CARTESIAN_POINT ( 'NONE',  ( 1.846868145590735200, -29.25000000136559564, -4.458734124999999437 ) ) ;
#4941=ORIENTED_EDGE ( 'NONE', *, *, #13234, .T. ) ;
#4952=ORIENTED_EDGE ( 'NONE', *, *, #11708, .F. ) ;
#4955=ORIENTED_EDGE ( 'NONE', *, *, #14391, .F. ) ;
#4967=CARTESIAN_POINT ( 'NONE',  ( -3.152801135295367096, -26.31250000136559564, -3.152801135295367541 ) ) ;
#4968=CARTESIAN_POINT ( 'NONE',  ( 1.846868145590736310, -21.62500000136559208, 4.458734124999997661 ) ) ;
#4975=CARTESIAN_POINT ( 'NONE',  ( -4.458734125000001214, -23.12500000136559564, 1.846868145590734089 ) ) ;
#4976=EDGE_CURVE ( 'NONE', #12106, #10564, #3297, .T. ) ;
#4980=EDGE_CURVE ( 'NONE', #3993, #11064, #1219, .T. ) ;
#4987=LINE ( 'NONE', #2879, #15459 ) ;
#4988=CARTESIAN_POINT ( 'NONE',  ( -8.190561711645485556E-16, -28.68750000136559564, 4.458734124999999437 ) ) ;
#4990=ORIENTED_EDGE ( 'NONE', *, *, #6750, .F. ) ;
#4995=CARTESIAN_POINT ( 'NONE',  ( 4.458734124999999437, -24.50000000136559564, 1.846868145590737864 ) ) ;
#4997=EDGE_LOOP ( 'NONE', ( #10338, #14838, #5170, #4840, #10897, #15620, #7765, #2828 ) ) ;
#5001=CARTESIAN_POINT ( 'NONE',  ( 0.000000000000000000, -20.00000000000000000, 0.000000000000000000 ) ) ;
#5004=CARTESIAN_POINT ( 'NONE',  ( -9.184850993605147944E-16, -30.25000000000000000, 5.000000000000000000 ) ) ;
#5007=CARTESIAN_POINT ( 'NONE',  ( -5.000000000000000888, -29.56250000273118417, 2.071067811865474617 ) ) ;
#5010=CARTESIAN_POINT ( 'NONE',  ( 4.458734124999997661, -28.50000000136559564, 1.846868145590737864 ) ) ;
#5019=EDGE_CURVE ( 'NONE', #4014, #7371, #6431, .T. ) ;
#5027=CARTESIAN_POINT ( 'NONE',  ( 5.000000000000000000, -24.00000000000000000, 0.000000000000000000 ) ) ;
#5030=DIRECTION ( 'NONE',  ( -0.000000000000000000, 1.000000000000000000, -0.000000000000000000 ) ) ;
#5032=( LENGTH_UNIT ( ) NAMED_UNIT ( * ) SI_UNIT ( .MILLI., .METRE. ) );
#5040=ADVANCED_FACE ( 'NONE', ( #12303 ), #12626, .T. ) ;
#5046=CARTESIAN_POINT ( 'NONE',  ( 5.000000000000000000, -27.12500000273118772, 0.000000000000000000 ) ) ;
#5050=CARTESIAN_POINT ( 'NONE',  ( -3.152801135295367985, -27.06250000136559564, 3.152801135295367096 ) ) ;
#5051=ORIENTED_EDGE ( 'NONE', *, *, #2929, .T. ) ;
#5052=FACE_OUTER_BOUND ( 'NONE', #5584, .T. ) ;
#5056=ORIENTED_EDGE ( 'NONE', *, *, #11652, .F. ) ;
#5059=CARTESIAN_POINT ( 'NONE',  ( -8.190561711645485556E-16, -23.93750000136559564, 4.458734124999999437 ) ) ;
#5064=LINE ( 'NONE', #2798, #5351 ) ;
#5072=CARTESIAN_POINT ( 'NONE',  ( -4.458734125000000326, -25.00000000136559564, -1.846868145590735644 ) ) ;
#5080=CARTESIAN_POINT ( 'NONE',  ( -4.458734125000000326, -25.00000000136559564, -1.846868145590735644 ) ) ;
#5081=DIRECTION ( 'NONE',  ( 0.000000000000000000, 0.000000000000000000, 1.000000000000000000 ) ) ;
#5089=DIRECTION ( 'NONE',  ( 0.000000000000000000, 1.000000000000000000, 0.000000000000000000 ) ) ;
#5090=CARTESIAN_POINT ( 'NONE',  ( 5.000000000000000888, -30.93750000000000355, -2.071067811865475505 ) ) ;
#5094=CARTESIAN_POINT ( 'NONE',  ( 3.535533905932736864, -27.25000000273118772, 3.535533905932738641 ) ) ;
#5096=CARTESIAN_POINT ( 'NONE',  ( 4.458734124999999437, -31.43750000136559564, 0.000000000000000000 ) ) ;
#5099=ORIENTED_EDGE ( 'NONE', *, *, #9786, .F. ) ;
#5102=ORIENTED_EDGE ( 'NONE', *, *, #9405, .F. ) ;
#5104=ORIENTED_EDGE ( 'NONE', *, *, #2974, .F. ) ;
#5105=LINE ( 'NONE', #3806, #15148 ) ;
#5108=CARTESIAN_POINT ( 'NONE',  ( -3.152801135295367096, -31.31250000136559564, -3.152801135295367541 ) ) ;
#5117=EDGE_CURVE ( 'NONE', #6271, #15920, #11582, .T. ) ;
#5125=ORIENTED_EDGE ( 'NONE', *, *, #3128, .T. ) ;
#5131=LINE ( 'NONE', #367, #8250 ) ;
#5135=AXIS2_PLACEMENT_3D ( 'NONE', #9093, #15064, #12867 ) ;
#5146=EDGE_LOOP ( 'NONE', ( #3777, #2829 ) ) ;
#5150=ORIENTED_EDGE ( 'NONE', *, *, #15232, .T. ) ;
#5153=DIRECTION ( 'NONE',  ( 0.000000000000000000, -1.000000000000000000, 0.000000000000000000 ) ) ;
#5159=CARTESIAN_POINT ( 'NONE',  ( 2.071067811865451080, -29.81249999999999645, -5.000000000000024869 ) ) ;
#5160=CARTESIAN_POINT ( 'NONE',  ( 5.000000000000000000, -29.06250000000000000, 2.071067811865478614 ) ) ;
#5161=CARTESIAN_POINT ( 'NONE',  ( -1.846868145590734756, -26.12500000136559564, -4.458734125000000326 ) ) ;
#5166=ORIENTED_EDGE ( 'NONE', *, *, #6898, .F. ) ;
#5168=CARTESIAN_POINT ( 'NONE',  ( -3.152801135295367985, -23.81250000136559564, 3.152801135295367096 ) ) ;
#5169=DIRECTION ( 'NONE',  ( 0.000000000000000000, -1.000000000000000000, 0.000000000000000000 ) ) ;
#5170=ORIENTED_EDGE ( 'NONE', *, *, #10229, .T. ) ;
#5175=CARTESIAN_POINT ( 'NONE',  ( -9.184850993605147944E-16, -31.25000000000000000, 5.000000000000000000 ) ) ;
#5177=PLANE ( 'NONE',  #8760 ) ;
#5178=CARTESIAN_POINT ( 'NONE',  ( 2.071067811865475505, -28.93750000273119483, -5.000000000000000888 ) ) ;
#5181=CARTESIAN_POINT ( 'NONE',  ( 5.000000000000000000, -24.12500000273118772, 0.000000000000000000 ) ) ;
#5188=CARTESIAN_POINT ( 'NONE',  ( 3.061616997868383141E-16, -24.87500000273118417, -5.000000000000000000 ) ) ;
#5191=CARTESIAN_POINT ( 'NONE',  ( 3.152801135295367541, -30.56250000136559564, -3.152801135295367541 ) ) ;
#5196=ORIENTED_EDGE ( 'NONE', *, *, #15736, .T. ) ;
#5206=CARTESIAN_POINT ( 'NONE',  ( 2.071067811865462183, -21.31250000273118772, 5.000000000000013323 ) ) ;
#5209=CARTESIAN_POINT ( 'NONE',  ( -5.000000000000000000, -23.50000000000000000, -6.123233995736766282E-16 ) ) ;
#5211=CARTESIAN_POINT ( 'NONE',  ( 4.458734124999997661, -21.75000000136559208, 1.846868145590737864 ) ) ;
#5212=VERTEX_POINT ( 'NONE', #5451 ) ;
#5220=LINE ( 'NONE', #6519, #15150 ) ;
#5222=CARTESIAN_POINT ( 'NONE',  ( -3.535533905932738641, -27.50000000273118772, 3.535533905932737309 ) ) ;
#5231=CARTESIAN_POINT ( 'NONE',  ( 3.152801135295366208, -22.56250000136559564, 3.152801135295367985 ) ) ;
#5236=ORIENTED_EDGE ( 'NONE', *, *, #3940, .T. ) ;
#5237=CARTESIAN_POINT ( 'NONE',  ( -1.846868145590737420, -30.00000000136559564, 4.458734124999999437 ) ) ;
#5248=CARTESIAN_POINT ( 'NONE',  ( 0.000000000000000000, -20.00000000000000000, 0.000000000000000000 ) ) ;
#5249=CARTESIAN_POINT ( 'NONE',  ( 3.535533905932738197, -30.87500000000000000, -3.535533905932738197 ) ) ;
#5252=CARTESIAN_POINT ( 'NONE',  ( 5.000000000000000888, -23.06250000273118417, -2.071067811865475505 ) ) ;
#5254=CARTESIAN_POINT ( 'NONE',  ( -4.458734124999999437, -30.93750000136559564, -5.460374474430324690E-16 ) ) ;
#5281=DIRECTION ( 'NONE',  ( 0.000000000000000000, 1.000000000000000000, 0.000000000000000000 ) ) ;
#5296=EDGE_LOOP ( 'NONE', ( #5166, #15581, #985, #9163 ) ) ;
#5298=EDGE_CURVE ( 'NONE', #13118, #3154, #12614, .T. ) ;
#5303=CARTESIAN_POINT ( 'NONE',  ( 6.123233995736766282E-16, -13.00000000000000178, -5.000000000000000000 ) ) ;
#5311=CARTESIAN_POINT ( 'NONE',  ( 4.458734124999999437, -22.43750000136559564, 0.000000000000000000 ) ) ;
#5315=CIRCLE ( 'NONE', #11495, 25.00000000000000000 ) ;
#5324=CARTESIAN_POINT ( 'NONE',  ( -4.458734124999999437, -31.18750000136559564, -5.460374474430324690E-16 ) ) ;
#5325=CARTESIAN_POINT ( 'NONE',  ( 3.061616997868383141E-16, -21.87500000273118772, -5.000000000000000000 ) ) ;
#5332=VECTOR ( 'NONE', #11612, 1000.000000000000000 ) ;
#5333=CARTESIAN_POINT ( 'NONE',  ( 3.535533905932736864, -29.12500000000000000, 3.535533905932738641 ) ) ;
#5336=DIRECTION ( 'NONE',  ( 1.000000000000000000, 0.000000000000000000, -1.239088197126290570E-16 ) ) ;
#5337=CARTESIAN_POINT ( 'NONE',  ( 3.535533905932738197, -23.00000000273118772, -3.535533905932738197 ) ) ;
#5339=CARTESIAN_POINT ( 'NONE',  ( 3.152801135295367541, -25.31250000136559564, -3.152801135295367541 ) ) ;
#5351=VECTOR ( 'NONE', #15085, 1000.000000000000000 ) ;
#5353=CARTESIAN_POINT ( 'NONE',  ( -1.846868145590734756, -30.37500000136559564, -4.458734125000000326 ) ) ;
#5361=EDGE_CURVE ( 'NONE', #10378, #8374, #4251, .T. ) ;
#5362=ORIENTED_EDGE ( 'NONE', *, *, #14391, .T. ) ;
#5365=CARTESIAN_POINT ( 'NONE',  ( -1.846868145590734756, -31.12500000136559564, -4.458734125000000326 ) ) ;
#5375=CARTESIAN_POINT ( 'NONE',  ( -3.152801135295367096, -23.31250000136559564, -3.152801135295367541 ) ) ;
#5377=FACE_OUTER_BOUND ( 'NONE', #11720, .T. ) ;
#5387=DIRECTION ( 'NONE',  ( 0.000000000000000000, 0.000000000000000000, 1.000000000000000000 ) ) ;
#5389=CYLINDRICAL_SURFACE ( 'NONE', #9665, 5.000000000000000000 ) ;
#5390=AXIS2_PLACEMENT_3D ( 'NONE', #4806, #6188, #3300 ) ;
#5392=DIRECTION ( 'NONE',  ( 0.000000000000000000, 0.000000000000000000, 1.000000000000000000 ) ) ;
#5394=DIRECTION ( 'NONE',  ( -0.000000000000000000, 1.000000000000000000, -0.000000000000000000 ) ) ;
#5403=DIRECTION ( 'NONE',  ( -1.000000000000000000, 0.000000000000000000, 1.239088197126290570E-16 ) ) ;
#5405=ORIENTED_EDGE ( 'NONE', *, *, #5117, .F. ) ;
#5406=VERTEX_POINT ( 'NONE', #3124 ) ;
#5407=CARTESIAN_POINT ( 'NONE',  ( -4.458734125000001214, -31.12500000136559564, 1.846868145590734089 ) ) ;
#5409=ORIENTED_EDGE ( 'NONE', *, *, #14328, .F. ) ;
#5418=CARTESIAN_POINT ( 'NONE',  ( -3.535533905932737309, -25.62500000000000355, -3.535533905932738197 ) ) ;
#5422=CARTESIAN_POINT ( 'NONE',  ( -2.071067811865478170, -24.43750000273119483, 5.000000000000000000 ) ) ;
#5424=CARTESIAN_POINT ( 'NONE',  ( -1.846868145590734756, -28.12500000136559564, -4.458734124999999437 ) ) ;
#5436=FACE_BOUND ( 'NONE', #5146, .T. ) ;
#5437=LINE ( 'NONE', #6489, #9850 ) ;
#5439=FACE_OUTER_BOUND ( 'NONE', #11297, .T. ) ;
#5444=CARTESIAN_POINT ( 'NONE',  ( -1.846868145590734756, -27.12500000136559564, -4.458734125000000326 ) ) ;
#5445=ORIENTED_EDGE ( 'NONE', *, *, #9103, .F. ) ;
#5448=EDGE_CURVE ( 'NONE', #14100, #9570, #2499, .T. ) ;
#5451=CARTESIAN_POINT ( 'NONE',  ( -24.26932219902319687, 40.00000000000000000, -5.999999999999984901 ) ) ;
#5455=CARTESIAN_POINT ( 'NONE',  ( -4.458734125000000326, -22.12500000136559564, 1.846868145590734089 ) ) ;
#5462=ORIENTED_EDGE ( 'NONE', *, *, #9108, .T. ) ;
#5468=CARTESIAN_POINT ( 'NONE',  ( 0.000000000000000000, -20.00000000000000000, 0.000000000000000000 ) ) ;
#5469=DIRECTION ( 'NONE',  ( -0.000000000000000000, -1.000000000000000000, -0.000000000000000000 ) ) ;
#5476=CARTESIAN_POINT ( 'NONE',  ( 4.458734124999999437, -22.50000000136559208, 1.846868145590737864 ) ) ;
#5483=CARTESIAN_POINT ( 'NONE',  ( -4.458734125000000326, -30.25000000136559564, -1.846868145590735644 ) ) ;
#5491=CARTESIAN_POINT ( 'NONE',  ( 2.071067811865475505, -26.81250000000000000, -5.000000000000000888 ) ) ;
#5495=CARTESIAN_POINT ( 'NONE',  ( -5.000000000000000000, -25.62500000273118417, -6.123233995736766282E-16 ) ) ;
#5497=CARTESIAN_POINT ( 'NONE',  ( -4.458734125000000326, -26.87500000136559919, 1.846868145590734089 ) ) ;
#5504=ORIENTED_EDGE ( 'NONE', *, *, #8743, .T. ) ;
#5511=CARTESIAN_POINT ( 'NONE',  ( -1.846868145590737420, -26.00000000136559564, 4.458734124999999437 ) ) ;
#5515=CARTESIAN_POINT ( 'NONE',  ( 5.000000000000000888, -31.93750000000000000, -2.071067811865475505 ) ) ;
#5522=EDGE_CURVE ( 'NONE', #10564, #8217, #974, .T. ) ;
#5535=CARTESIAN_POINT ( 'NONE',  ( -5.000000000000000888, -26.68750000273119127, -2.071067811865475949 ) ) ;
#5543=CARTESIAN_POINT ( 'NONE',  ( -5.000000000000000000, -30.50000000000000000, -6.123233995736766282E-16 ) ) ;
#5554=CARTESIAN_POINT ( 'NONE',  ( -1.846868145590737420, -21.75000000136559564, 4.458734124999999437 ) ) ;
#5557=CARTESIAN_POINT ( 'NONE',  ( 35.00000000000000000, 37.00000000000000000, 5.999999999999991118 ) ) ;
#5564=CARTESIAN_POINT ( 'NONE',  ( 4.458734125000000326, -25.62500000136559564, -1.846868145590734978 ) ) ;
#5572=CARTESIAN_POINT ( 'NONE',  ( 3.535533905932736864, -25.12500000000000000, 3.535533905932738641 ) ) ;
#5577=CARTESIAN_POINT ( 'NONE',  ( 2.071067811865475505, -25.93750000273118772, -5.000000000000000888 ) ) ;
#5581=CARTESIAN_POINT ( 'NONE',  ( 1.846868145590736310, -24.62500000136559564, 4.458734124999997661 ) ) ;
#5583=ORIENTED_EDGE ( 'NONE', *, *, #5117, .T. ) ;
#5584=EDGE_LOOP ( 'NONE', ( #7819, #735, #15524, #7576 ) ) ;
#5591=CARTESIAN_POINT ( 'NONE',  ( 2.730187237215162345E-16, -29.43750000136559208, -4.458734124999999437 ) ) ;
#5595=DIRECTION ( 'NONE',  ( 0.8660254037844410391, -0.4999999999999958367, 0.000000000000000000 ) ) ;
#5596=CARTESIAN_POINT ( 'NONE',  ( 5.000000000000000000, -32.00000000000000000, 0.000000000000000000 ) ) ;
#5603=ADVANCED_FACE ( 'NONE', ( #5439 ), #3002, .T. ) ;
#5604=AXIS2_PLACEMENT_3D ( 'NONE', #8459, #8539, #10943 ) ;
#5606=CARTESIAN_POINT ( 'NONE',  ( -5.000000000000000888, -27.68750000273119127, -2.071067811865475949 ) ) ;
#5628=CARTESIAN_POINT ( 'NONE',  ( -9.184850993605147944E-16, -31.25000000000000000, 5.000000000000000000 ) ) ;
#5629=CARTESIAN_POINT ( 'NONE',  ( -5.000000000000000888, -25.43750000000000355, 2.071067811865474617 ) ) ;
#5636=CARTESIAN_POINT ( 'NONE',  ( 2.730187237215162345E-16, -30.43750000136559564, -4.458734124999999437 ) ) ;
#5638=ORIENTED_EDGE ( 'NONE', *, *, #15597, .T. ) ;
#5645=CARTESIAN_POINT ( 'NONE',  ( -3.152801135295367985, -28.06250000136559564, 3.152801135295367096 ) ) ;
#5654=CARTESIAN_POINT ( 'NONE',  ( -9.184850993605147944E-16, -26.25000000000000355, 5.000000000000000000 ) ) ;
#5658=CARTESIAN_POINT ( 'NONE',  ( -4.458734124999999437, -30.93750000136559564, -5.460374474430324690E-16 ) ) ;
#5661=CARTESIAN_POINT ( 'NONE',  ( -1.846868145590737420, -27.75000000136559564, 4.458734124999997661 ) ) ;
#5672=CARTESIAN_POINT ( 'NONE',  ( -4.458734125000001214, -29.12500000136559919, 1.846868145590734089 ) ) ;
#5690=CARTESIAN_POINT ( 'NONE',  ( -35.00000000000000000, 40.00000000000000000, 2.649999999999992806 ) ) ;
#5694=DIRECTION ( 'NONE',  ( 0.000000000000000000, 0.000000000000000000, -1.000000000000000000 ) ) ;
#5696=CARTESIAN_POINT ( 'NONE',  ( 5.000000000000000888, -26.93750000000000355, -2.071067811865475505 ) ) ;
#5699=CARTESIAN_POINT ( 'NONE',  ( 5.000000000000000888, -23.06250000273119127, -2.071067811865475505 ) ) ;
#5706=CARTESIAN_POINT ( 'NONE',  ( 3.535533905932736864, -23.12500000000000000, 3.535533905932738641 ) ) ;
#5710=CARTESIAN_POINT ( 'NONE',  ( 2.730187237215162345E-16, -31.43750000136559564, -4.458734124999999437 ) ) ;
#5716=CARTESIAN_POINT ( 'NONE',  ( -3.152801135295367096, -26.31250000136559564, -3.152801135295367541 ) ) ;
#5717=CARTESIAN_POINT ( 'NONE',  ( 5.000000000000000000, -31.56250000136559564, 0.000000000000000000 ) ) ;
#5724=CARTESIAN_POINT ( 'NONE',  ( 3.535533905932738197, -24.87500000000000000, -3.535533905932738197 ) ) ;
#5728=CARTESIAN_POINT ( 'NONE',  ( 1.846868145590735200, -29.25000000136559564, -4.458734125000000326 ) ) ;
#5729=ORIENTED_EDGE ( 'NONE', *, *, #15736, .F. ) ;
#5730=CARTESIAN_POINT ( 'NONE',  ( 2.730187237215162345E-16, -24.18750000136559564, -4.458734124999999437 ) ) ;
#5735=CARTESIAN_POINT ( 'NONE',  ( 3.152801135295366208, -28.56250000136559564, 3.152801135295367985 ) ) ;
#5740=( BOUNDED_CURVE ( )  B_SPLINE_CURVE ( 2, ( #14419, #14654, #4711, #3345, #13183, #15870, #15722, #2118, #2285 ),
 .UNSPECIFIED., .F., .F. ) 
 B_SPLINE_CURVE_WITH_KNOTS ( ( 3, 2, 2, 2, 3 ),
 ( 0.8750000000000000000, 0.8874999999999999556, 0.8999999999999999112, 0.9124999999999998668, 0.9249999999999998224 ),
 .UNSPECIFIED. ) 
 CURVE ( )  GEOMETRIC_REPRESENTATION_ITEM ( )  RATIONAL_B_SPLINE_CURVE ( ( 1.000000000000000000, 0.9238795325112867385, 1.000000000000000000, 0.9238795325112867385, 1.000000000000000000, 0.9238795325112867385, 1.000000000000000000, 0.9238795325112880708, 0.9999999999999986677 ) ) 
 REPRESENTATION_ITEM ( '' )  );
#5744=CARTESIAN_POINT ( 'NONE',  ( -3.152801135295367096, -29.31250000136559564, -3.152801135295367541 ) ) ;
#5746=LINE ( 'NONE', #8111, #9281 ) ;
#5763=CARTESIAN_POINT ( 'NONE',  ( 2.071067811865462183, -25.18750000000000355, 5.000000000000013323 ) ) ;
#5765=CYLINDRICAL_SURFACE ( 'NONE', #990, 5.999999999999991118 ) ;
#5772=CARTESIAN_POINT ( 'NONE',  ( 3.061616997868383141E-16, -22.87500000273118772, -5.000000000000000000 ) ) ;
#5778=CARTESIAN_POINT ( 'NONE',  ( 0.000000000000000000, -11.00000000000000178, -6.000000000000000888 ) ) ;
#5782=CARTESIAN_POINT ( 'NONE',  ( 3.061616997868383141E-16, -22.87500000273118772, -5.000000000000000000 ) ) ;
#5783=CARTESIAN_POINT ( 'NONE',  ( 3.152801135295366208, -27.81250000136559564, 3.152801135295367985 ) ) ;
#5792=CARTESIAN_POINT ( 'NONE',  ( -4.458734125000000326, -26.25000000136559208, -1.846868145590735644 ) ) ;
#5793=CARTESIAN_POINT ( 'NONE',  ( 3.061616997868383043E-15, 40.00000000000000000, -25.00000000000000000 ) ) ;
#5801=CARTESIAN_POINT ( 'NONE',  ( 5.809475019311125976, -13.00000000000000178, 1.500000000000000000 ) ) ;
#5802=EDGE_CURVE ( 'NONE', #2074, #9076, #14799, .T. ) ;
#5803=LINE ( 'NONE', #6720, #2539 ) ;
#5804=EDGE_CURVE ( 'NONE', #7371, #79, #464, .T. ) ;
#5805=CARTESIAN_POINT ( 'NONE',  ( 1.846868145590736310, -30.62500000136559208, 4.458734124999999437 ) ) ;
#5809=CARTESIAN_POINT ( 'NONE',  ( -1.846868145590734756, -24.12500000136559919, -4.458734124999999437 ) ) ;
#5815=CARTESIAN_POINT ( 'NONE',  ( 4.458734124999999437, -29.50000000136559564, 1.846868145590737864 ) ) ;
#5820=CARTESIAN_POINT ( 'NONE',  ( 2.071067811865505259, -22.18749999999999645, 4.999999999999970690 ) ) ;
#5823=CARTESIAN_POINT ( 'NONE',  ( 3.152801135295366208, -27.81250000136559564, 3.152801135295367985 ) ) ;
#5828=DIRECTION ( 'NONE',  ( -1.000000000000000000, 0.000000000000000000, 0.000000000000000000 ) ) ;
#5831=VECTOR ( 'NONE', #3754, 1000.000000000000000 ) ;
#5844=ADVANCED_FACE ( 'NONE', ( #13075 ), #3226, .T. ) ;
#5847=CARTESIAN_POINT ( 'NONE',  ( 7.347880794884120722E-16, -11.00000000000000178, 6.000000000000000888 ) ) ;
#5850=CARTESIAN_POINT ( 'NONE',  ( -3.535533905932737309, -22.62500000000000000, -3.535533905932738197 ) ) ;
#5858=CARTESIAN_POINT ( 'NONE',  ( -3.535533905932738641, -23.50000000273118772, 3.535533905932737309 ) ) ;
#5860=PLANE ( 'NONE',  #15877 ) ;
#5862=AXIS2_PLACEMENT_3D ( 'NONE', #9888, #7397, #7482 ) ;
#5863=CARTESIAN_POINT ( 'NONE',  ( -9.184850993605147944E-16, -24.37500000273118772, 5.000000000000000000 ) ) ;
#5869=CARTESIAN_POINT ( 'NONE',  ( -1.846868145590734756, -31.37500000136559564, -4.458734124999999437 ) ) ;
#5877=CARTESIAN_POINT ( 'NONE',  ( 1.846868145590735200, -26.50000000136559208, -4.458734125000000326 ) ) ;
#5879=CARTESIAN_POINT ( 'NONE',  ( 3.061616997868383141E-16, -25.87500000273118417, -5.000000000000000000 ) ) ;
#5881=AXIS2_PLACEMENT_3D ( 'NONE', #15072, #3914, #15158 ) ;
#5884=CARTESIAN_POINT ( 'NONE',  ( -5.000000000000000000, -22.50000000000000000, -6.123233995736766282E-16 ) ) ;
#5886=CARTESIAN_POINT ( 'NONE',  ( -2.071067811865492381, -21.43750000273118772, 4.999999999999985789 ) ) ;
#5889=CARTESIAN_POINT ( 'NONE',  ( 1.846868145590735200, -31.25000000136559564, -4.458734125000000326 ) ) ;
#5897=AXIS2_PLACEMENT_3D ( 'NONE', #12664, #1604, #2651 ) ;
#5898=CARTESIAN_POINT ( 'NONE',  ( -1.846868145590737420, -29.75000000136559564, 4.458734124999999437 ) ) ;
#5902=ADVANCED_FACE ( 'NONE', ( #455, #5377 ), #15245, .F. ) ;
#5904=VECTOR ( 'NONE', #15013, 1000.000000000000000 ) ;
#5911=CARTESIAN_POINT ( 'NONE',  ( -3.152801135295367096, -23.31250000136559564, -3.152801135295367541 ) ) ;
#5915=CARTESIAN_POINT ( 'NONE',  ( -2.071067811865478170, -30.43750000273118417, 5.000000000000000000 ) ) ;
#5921=CARTESIAN_POINT ( 'NONE',  ( 0.000000000000000000, 20.00000000000000000, 0.000000000000000000 ) ) ;
#5922=ORIENTED_EDGE ( 'NONE', *, *, #713, .F. ) ;
#5924=CARTESIAN_POINT ( 'NONE',  ( -3.535533905932737309, -26.62500000000000000, -3.535533905932738197 ) ) ;
#5931=DIRECTION ( 'NONE',  ( 0.000000000000000000, -1.000000000000000000, 0.000000000000000000 ) ) ;
#5951=CARTESIAN_POINT ( 'NONE',  ( -4.458734125000000326, -30.12500000136559564, 1.846868145590734089 ) ) ;
#5958=EDGE_LOOP ( 'NONE', ( #10585, #7409, #11335, #5236 ) ) ;
#5961=ADVANCED_FACE ( 'NONE', ( #5052 ), #7814, .T. ) ;
#5970=CARTESIAN_POINT ( 'NONE',  ( -3.152801135295367985, -29.81250000136559208, 3.152801135295367096 ) ) ;
#5977=CARTESIAN_POINT ( 'NONE',  ( -3.152801135295367096, -27.06250000136559564, -3.152801135295367541 ) ) ;
#5984=CARTESIAN_POINT ( 'NONE',  ( 1.846868145590735200, -23.50000000136559564, -4.458734125000000326 ) ) ;
#5987=CARTESIAN_POINT ( 'NONE',  ( -5.000000000000000888, -30.56250000273118417, 2.071067811865474617 ) ) ;
#5995=DIRECTION ( 'NONE',  ( 0.000000000000000000, 0.000000000000000000, 1.000000000000000000 ) ) ;
#6014=ORIENTED_EDGE ( 'NONE', *, *, #2929, .F. ) ;
#6017=DIRECTION ( 'NONE',  ( 0.000000000000000000, 0.000000000000000000, 1.000000000000000000 ) ) ;
#6022=CARTESIAN_POINT ( 'NONE',  ( 24.26932219902320043, 37.00000000000000000, 5.999999999999992895 ) ) ;
#6023=LINE ( 'NONE', #9575, #10038 ) ;
#6028=CARTESIAN_POINT ( 'NONE',  ( 4.458734124999999437, -25.62500000136559564, -1.846868145590734978 ) ) ;
#6031=CARTESIAN_POINT ( 'NONE',  ( 0.000000000000000000, 20.00000000000000000, 0.000000000000000000 ) ) ;
#6037=CARTESIAN_POINT ( 'NONE',  ( 1.846868145590736310, -24.87500000136559919, 4.458734124999999437 ) ) ;
#6039=CARTESIAN_POINT ( 'NONE',  ( 5.000000000000000000, -30.12500000273118417, 0.000000000000000000 ) ) ;
#6042=CARTESIAN_POINT ( 'NONE',  ( -5.000000000000000000, -23.50000000000000000, -6.123233995736766282E-16 ) ) ;
#6045=CARTESIAN_POINT ( 'NONE',  ( -5.000000000000000888, -27.43750000000000355, 2.071067811865474617 ) ) ;
#6046=CARTESIAN_POINT ( 'NONE',  ( 4.458734125000000326, -27.37500000136559564, -1.846868145590734978 ) ) ;
#6055=CARTESIAN_POINT ( 'NONE',  ( -8.190561711645485556E-16, -25.68750000136559564, 4.458734124999999437 ) ) ;
#6060=CARTESIAN_POINT ( 'NONE',  ( -9.184850993605147944E-16, -22.25000000000000000, 4.999999999999999112 ) ) ;
#6063=CARTESIAN_POINT ( 'NONE',  ( -8.190561711645485556E-16, -23.93750000136559564, 4.458734124999999437 ) ) ;
#6066=CARTESIAN_POINT ( 'NONE',  ( 5.000000000000000888, -28.06250000273118772, -2.071067811865475505 ) ) ;
#6073=CARTESIAN_POINT ( 'NONE',  ( 0.000000000000000000, -11.00000000000000178, 5.000000000000000000 ) ) ;
#6076=EDGE_LOOP ( 'NONE', ( #695, #654, #9307, #12793 ) ) ;
#6078=AXIS2_PLACEMENT_3D ( 'NONE', #4804, #11028, #14502 ) ;
#6083=AXIS2_PLACEMENT_3D ( 'NONE', #417, #7854, #7782 ) ;
#6097=EDGE_CURVE ( 'NONE', #3419, #10619, #9180, .T. ) ;
#6099=CARTESIAN_POINT ( 'NONE',  ( -5.000000000000000000, -29.50000000000000355, -6.123233995736766282E-16 ) ) ;
#6103=UNCERTAINTY_MEASURE_WITH_UNIT (LENGTH_MEASURE( 1.000000000000000082E-05 ), #10053, 'distance_accuracy_value', 'NONE');
#6104=CARTESIAN_POINT ( 'NONE',  ( -3.535533905932738641, -29.50000000273118417, 3.535533905932737309 ) ) ;
#6107=VECTOR ( 'NONE', #12527, 1000.000000000000000 ) ;
#6109=CARTESIAN_POINT ( 'NONE',  ( 3.152801135295367541, -24.56250000136559564, -3.152801135295367541 ) ) ;
#6110=CARTESIAN_POINT ( 'NONE',  ( -4.458734124999999437, -23.93750000136559564, -5.460374474430324690E-16 ) ) ;
#6115=CARTESIAN_POINT ( 'NONE',  ( 3.152801135295366208, -24.81250000136559564, 3.152801135295367985 ) ) ;
#6119=CARTESIAN_POINT ( 'NONE',  ( 4.458734124999999437, -24.75000000136559564, 1.846868145590737864 ) ) ;
#6120=CARTESIAN_POINT ( 'NONE',  ( -5.000000000000000888, -23.56250000273118772, 2.071067811865474617 ) ) ;
#6121=CARTESIAN_POINT ( 'NONE',  ( 3.061616997868383141E-16, -27.87500000273118772, -5.000000000000000000 ) ) ;
#6132=CARTESIAN_POINT ( 'NONE',  ( -3.152801135295367096, -27.06250000136559564, -3.152801135295367541 ) ) ;
#6134=ORIENTED_EDGE ( 'NONE', *, *, #13573, .T. ) ;
#6136=ORIENTED_EDGE ( 'NONE', *, *, #3940, .F. ) ;
#6140=CARTESIAN_POINT ( 'NONE',  ( 1.846868145590736310, -26.62500000136559564, 4.458734124999999437 ) ) ;
#6145=PLANE ( 'NONE',  #926 ) ;
#6152=CARTESIAN_POINT ( 'NONE',  ( -3.152801135295367985, -24.06250000136559564, 3.152801135295367096 ) ) ;
#6155=CARTESIAN_POINT ( 'NONE',  ( 5.000000000000000000, -30.18750000273118772, 2.071067811865478614 ) ) ;
#6158=CARTESIAN_POINT ( 'NONE',  ( 4.458734124999997661, -29.50000000136559564, 1.846868145590737864 ) ) ;
#6167=ADVANCED_FACE ( 'NONE', ( #9411 ), #5765, .T. ) ;
#6171=AXIS2_PLACEMENT_3D ( 'NONE', #2136, #15653, #15740 ) ;
#6175=DIRECTION ( 'NONE',  ( -0.000000000000000000, -1.000000000000000000, -0.000000000000000000 ) ) ;
#6188=DIRECTION ( 'NONE',  ( 0.000000000000000000, 1.000000000000000000, 0.000000000000000000 ) ) ;
#6196=CARTESIAN_POINT ( 'NONE',  ( -1.846868145590737420, -27.00000000136559564, 4.458734124999997661 ) ) ;
#6197=CARTESIAN_POINT ( 'NONE',  ( -3.152801135295367985, -21.81250000136559208, 3.152801135295367096 ) ) ;
#6206=CARTESIAN_POINT ( 'NONE',  ( 5.000000000000000000, -31.12500000273118772, 0.000000000000000000 ) ) ;
#6215=CARTESIAN_POINT ( 'NONE',  ( 3.152801135295367541, -25.31250000136559564, -3.152801135295367541 ) ) ;
#6224=CARTESIAN_POINT ( 'NONE',  ( -3.152801135295367096, -23.06250000136559564, -3.152801135295367541 ) ) ;
#6231=CARTESIAN_POINT ( 'NONE',  ( -4.458734124999999437, -24.18750000136559564, -5.460374474430324690E-16 ) ) ;
#6234=CARTESIAN_POINT ( 'NONE',  ( 5.000000000000000888, -27.06250000273118772, -2.071067811865475505 ) ) ;
#6236=CARTESIAN_POINT ( 'NONE',  ( -3.152801135295367985, -28.81250000136559564, 3.152801135295367096 ) ) ;
#6239=ORIENTED_EDGE ( 'NONE', *, *, #11945, .T. ) ;
#6244=EDGE_LOOP ( 'NONE', ( #14571, #13955, #6467, #3372 ) ) ;
#6248=AXIS2_PLACEMENT_3D ( 'NONE', #9547, #10611, #13004 ) ;
#6252=CARTESIAN_POINT ( 'NONE',  ( -9.184850993605147944E-16, -24.25000000000000000, 5.000000000000000000 ) ) ;
#6270=CARTESIAN_POINT ( 'NONE',  ( -8.190561711645485556E-16, -23.93750000136559564, 4.458734124999999437 ) ) ;
#6271=VERTEX_POINT ( 'NONE', #9718 ) ;
#6274=AXIS2_PLACEMENT_3D ( 'NONE', #11327, #12521, #2912 ) ;
#6281=CARTESIAN_POINT ( 'NONE',  ( 3.061616997868383141E-16, -30.87500000273118772, -5.000000000000000000 ) ) ;
#6286=EDGE_CURVE ( 'NONE', #10095, #13586, #2608, .T. ) ;
#6293=CARTESIAN_POINT ( 'NONE',  ( 4.458734125000000326, -25.37500000136559919, -1.846868145590734978 ) ) ;
#6301=CARTESIAN_POINT ( 'NONE',  ( 4.458734125000000326, -26.37500000136559564, -1.846868145590734978 ) ) ;
#6310=CARTESIAN_POINT ( 'NONE',  ( 3.061616997868383141E-16, -31.75000000000000000, -5.000000000000000000 ) ) ;
#6313=CARTESIAN_POINT ( 'NONE',  ( 3.061616997868383141E-16, -28.87500000273118772, -5.000000000000000000 ) ) ;
#6318=ORIENTED_EDGE ( 'NONE', *, *, #1179, .F. ) ;
#6322=DIRECTION ( 'NONE',  ( 0.000000000000000000, 1.000000000000000000, 0.000000000000000000 ) ) ;
#6327=CARTESIAN_POINT ( 'NONE',  ( 35.00000000000000000, 37.00000000000000000, -8.572527594031472993E-15 ) ) ;
#6339=ORIENTED_EDGE ( 'NONE', *, *, #4976, .T. ) ;
#6346=CARTESIAN_POINT ( 'NONE',  ( 5.000000000000000888, -27.06250000273118772, -2.071067811865475505 ) ) ;
#6349=CARTESIAN_POINT ( 'NONE',  ( -5.000000000000000888, -23.56250000000000000, -2.071067811865475949 ) ) ;
#6351=CARTESIAN_POINT ( 'NONE',  ( -1.846868145590734756, -22.37500000136559564, -4.458734124999999437 ) ) ;
#6357=VERTEX_POINT ( 'NONE', #13343 ) ;
#6360=VECTOR ( 'NONE', #4237, 1000.000000000000000 ) ;
#6361=ORIENTED_EDGE ( 'NONE', *, *, #5361, .T. ) ;
#6363=FACE_OUTER_BOUND ( 'NONE', #8684, .T. ) ;
#6372=CARTESIAN_POINT ( 'NONE',  ( 5.000000000000000000, -30.00000000000000000, 0.000000000000000000 ) ) ;
#6374=CARTESIAN_POINT ( 'NONE',  ( 1.846868145590736310, -26.62500000136559564, 4.458734124999999437 ) ) ;
#6379=ORIENTED_EDGE ( 'NONE', *, *, #11874, .F. ) ;
#6381=CARTESIAN_POINT ( 'NONE',  ( -1.846868145590734756, -26.12500000136559564, -4.458734125000000326 ) ) ;
#6387=PRODUCT_DEFINITION_FORMATION_WITH_SPECIFIED_SOURCE ( 'ANY', '', #4208, .NOT_KNOWN. ) ;
#6391=CARTESIAN_POINT ( 'NONE',  ( -2.071067811865475061, -31.68750000000000000, -5.000000000000000888 ) ) ;
#6394=CARTESIAN_POINT ( 'NONE',  ( 2.071067811865476394, -30.31250000273118772, 5.000000000000000000 ) ) ;
#6396=CARTESIAN_POINT ( 'NONE',  ( 2.071067811865475505, -23.93750000273119127, -5.000000000000000888 ) ) ;
#6406=ORIENTED_EDGE ( 'NONE', *, *, #8377, .T. ) ;
#6423=ADVANCED_FACE ( 'NONE', ( #3895 ), #13916, .T. ) ;
#6428=VECTOR ( 'NONE', #4534, 1000.000000000000000 ) ;
#6430=CARTESIAN_POINT ( 'NONE',  ( -5.000000000000000888, -28.56250000273119127, 2.071067811865474617 ) ) ;
#6431=LINE ( 'NONE', #1320, #721 ) ;
#6446=EDGE_CURVE ( 'NONE', #2074, #2190, #110, .T. ) ;
#6450=CARTESIAN_POINT ( 'NONE',  ( -5.000000000000000888, -27.56250000273118772, 2.071067811865474617 ) ) ;
#6457=CARTESIAN_POINT ( 'NONE',  ( -4.458734124999999437, -21.93750000136559208, -5.460374474430324690E-16 ) ) ;
#6465=CARTESIAN_POINT ( 'NONE',  ( 4.458734125000000326, -30.62500000136559208, -1.846868145590734978 ) ) ;
#6466=DIRECTION ( 'NONE',  ( -0.000000000000000000, 1.000000000000000000, -0.000000000000000000 ) ) ;
#6467=ORIENTED_EDGE ( 'NONE', *, *, #12564, .T. ) ;
#6468=CARTESIAN_POINT ( 'NONE',  ( 3.061616997868383141E-16, -28.75000000000000000, -5.000000000000000000 ) ) ;
#6472=CARTESIAN_POINT ( 'NONE',  ( -5.000000000000000000, -31.50000000000000000, -6.123233995736766282E-16 ) ) ;
#6475=CARTESIAN_POINT ( 'NONE',  ( -5.000000000000000000, -23.62500000273118772, -6.123233995736766282E-16 ) ) ;
#6477=CARTESIAN_POINT ( 'NONE',  ( 1.846868145590735200, -31.25000000136559564, -4.458734124999999437 ) ) ;
#6482=ORIENTED_EDGE ( 'NONE', *, *, #5804, .T. ) ;
#6485=CARTESIAN_POINT ( 'NONE',  ( 0.000000000000000000, -20.00000000000000000, 5.000000000000000000 ) ) ;
#6488=DIRECTION ( 'NONE',  ( -0.000000000000000000, 1.000000000000000000, -0.000000000000000000 ) ) ;
#6489=CARTESIAN_POINT ( 'NONE',  ( 35.00000000000000000, 37.00000000000000000, 5.999999999999991118 ) ) ;
#6494=DIRECTION ( 'NONE',  ( 1.000000000000000000, 0.000000000000000000, -0.000000000000000000 ) ) ;
#6509=CARTESIAN_POINT ( 'NONE',  ( -2.071067811865478170, -23.31249999999999645, 5.000000000000000000 ) ) ;
#6511=CARTESIAN_POINT ( 'NONE',  ( -3.152801135295367985, -22.06250000136559564, 3.152801135295367096 ) ) ;
#6519=CARTESIAN_POINT ( 'NONE',  ( 6.123233995736766282E-16, -20.00000000000000000, -5.000000000000000000 ) ) ;
#6530=CARTESIAN_POINT ( 'NONE',  ( 2.071067811865462183, -29.18749999999999645, 5.000000000000013323 ) ) ;
#6531=CARTESIAN_POINT ( 'NONE',  ( -1.846868145590734756, -24.12500000136559919, -4.458734125000000326 ) ) ;
#6537=CARTESIAN_POINT ( 'NONE',  ( 3.152801135295366208, -22.56250000136559564, 3.152801135295367985 ) ) ;
#6547=CARTESIAN_POINT ( 'NONE',  ( 5.000000000000000000, -28.00000000000000000, 0.000000000000000000 ) ) ;
#6550=CARTESIAN_POINT ( 'NONE',  ( -5.000000000000000888, -22.56250000273118772, 2.071067811865474617 ) ) ;
#6553=CARTESIAN_POINT ( 'NONE',  ( -4.458734125000000326, -27.87500000136559564, 1.846868145590734089 ) ) ;
#6557=EDGE_LOOP ( 'NONE', ( #1004, #5462 ) ) ;
#6567=CARTESIAN_POINT ( 'NONE',  ( 3.061616997868383141E-16, -31.75000000000000000, -5.000000000000000000 ) ) ;
#6572=CARTESIAN_POINT ( 'NONE',  ( 2.730187237215162345E-16, -31.18750000136559564, -4.458734124999999437 ) ) ;
#6574=ORIENTED_EDGE ( 'NONE', *, *, #14920, .F. ) ;
#6585=SURFACE_SIDE_STYLE ('',( #4401 ) ) ;
#6591=CARTESIAN_POINT ( 'NONE',  ( 3.061616997868383141E-16, -26.87500000273118772, -5.000000000000000000 ) ) ;
#6593=CARTESIAN_POINT ( 'NONE',  ( -35.00000000000000000, 40.00000000000000000, 6.000000000000000000 ) ) ;
#6594=ORIENTED_EDGE ( 'NONE', *, *, #14209, .T. ) ;
#6595=ORIENTED_EDGE ( 'NONE', *, *, #335, .F. ) ;
#6605=DIRECTION ( 'NONE',  ( 0.000000000000000000, 1.000000000000000000, 0.000000000000000000 ) ) ;
#6609=DIRECTION ( 'NONE',  ( -0.000000000000000000, 1.000000000000000000, -0.000000000000000000 ) ) ;
#6619=CARTESIAN_POINT ( 'NONE',  ( -1.846868145590734756, -31.37500000136559564, -4.458734125000000326 ) ) ;
#6628=DIRECTION ( 'NONE',  ( -0.000000000000000000, 1.000000000000000000, -0.000000000000000000 ) ) ;
#6629=CARTESIAN_POINT ( 'NONE',  ( -2.071067811865475061, -27.68750000000000355, -5.000000000000000888 ) ) ;
#6634=CARTESIAN_POINT ( 'NONE',  ( -9.184850993605147944E-16, -25.37500000273118417, 5.000000000000000000 ) ) ;
#6636=CARTESIAN_POINT ( 'NONE',  ( 2.730187237215162345E-16, -28.18750000136559564, -4.458734124999999437 ) ) ;
#6638=ORIENTED_EDGE ( 'NONE', *, *, #250, .T. ) ;
#6640=EDGE_LOOP ( 'NONE', ( #14553, #9288, #5104, #6704 ) ) ;
#6649=CYLINDRICAL_SURFACE ( 'NONE', #7162, 2.649999999999992806 ) ;
#6650=( BOUNDED_CURVE ( )  B_SPLINE_CURVE ( 2, ( #9277, #14200, #3123, #8067, #704, #5629, #10574, #15499, #4649 ),
 .UNSPECIFIED., .F., .F. ) 
 B_SPLINE_CURVE_WITH_KNOTS ( ( 3, 2, 2, 2, 3 ),
 ( 0.6249999999999998890, 0.6374999999999998446, 0.6499999999999999112, 0.6624999999999998668, 0.6749999999999999334 ),
 .UNSPECIFIED. ) 
 CURVE ( )  GEOMETRIC_REPRESENTATION_ITEM ( )  RATIONAL_B_SPLINE_CURVE ( ( 1.000000000000000666, 0.9238795325112860723, 1.000000000000000000, 0.9238795325112867385, 1.000000000000000000, 0.9238795325112867385, 1.000000000000000000, 0.9238795325112874046, 0.9999999999999993339 ) ) 
 REPRESENTATION_ITEM ( '' )  );
#6653=CARTESIAN_POINT ( 'NONE',  ( -3.152801135295367985, -30.06250000136559564, 3.152801135295367096 ) ) ;
#6659=( NAMED_UNIT ( * ) PLANE_ANGLE_UNIT ( ) SI_UNIT ( $, .RADIAN. ) );
#6661=VERTEX_POINT ( 'NONE', #1204 ) ;
#6664=CARTESIAN_POINT ( 'NONE',  ( 3.152801135295366208, -27.56250000136559564, 3.152801135295367985 ) ) ;
#6666=VERTEX_POINT ( 'NONE', #4189 ) ;
#6669=FACE_OUTER_BOUND ( 'NONE', #13874, .T. ) ;
#6677=PLANE ( 'NONE',  #8243 ) ;
#6678=CARTESIAN_POINT ( 'NONE',  ( -4.458734124999999437, -23.25000000136559564, -1.846868145590735644 ) ) ;
#6683=CARTESIAN_POINT ( 'NONE',  ( -2.071067811865482167, -26.81250000273118417, -4.999999999999992895 ) ) ;
#6697=ADVANCED_FACE ( 'NONE', ( #12741 ), #1443, .F. ) ;
#6701=CARTESIAN_POINT ( 'NONE',  ( 2.730187237215162345E-16, -23.18750000136559564, -4.458734124999999437 ) ) ;
#6702=AXIS2_PLACEMENT_3D ( 'NONE', #11940, #1195, #12019 ) ;
#6704=ORIENTED_EDGE ( 'NONE', *, *, #2866, .F. ) ;
#6709=CARTESIAN_POINT ( 'NONE',  ( -8.190561711645485556E-16, -30.93750000136559564, 4.458734124999999437 ) ) ;
#6717=CARTESIAN_POINT ( 'NONE',  ( 5.000000000000000888, -25.93750000000000355, -2.071067811865475505 ) ) ;
#6719=DIRECTION ( 'NONE',  ( -1.239088197126290570E-16, 0.000000000000000000, -1.000000000000000000 ) ) ;
#6720=CARTESIAN_POINT ( 'NONE',  ( 35.00000000000000000, 37.00000000000000000, -2.650000000000001243 ) ) ;
#6721=EDGE_CURVE ( 'NONE', #349, #12690, #3830, .T. ) ;
#6722=CARTESIAN_POINT ( 'NONE',  ( -5.000000000000000888, -24.56250000273118772, 2.071067811865474617 ) ) ;
#6725=CARTESIAN_POINT ( 'NONE',  ( 3.152801135295366208, -24.56250000136559564, 3.152801135295367985 ) ) ;
#6726=CARTESIAN_POINT ( 'NONE',  ( -9.184850993605147944E-16, -22.37500000273118417, 5.000000000000000000 ) ) ;
#6735=CARTESIAN_POINT ( 'NONE',  ( -4.458734125000001214, -26.12500000136559919, 1.846868145590734089 ) ) ;
#6738=EDGE_CURVE ( 'NONE', #14678, #13455, #12341, .T. ) ;
#6739=DIRECTION ( 'NONE',  ( -0.000000000000000000, 1.000000000000000000, -0.000000000000000000 ) ) ;
#6750=EDGE_CURVE ( 'NONE', #8728, #15000, #1294, .T. ) ;
#6753=DIRECTION ( 'NONE',  ( -1.000000000000000000, 0.000000000000000000, -0.000000000000000000 ) ) ;
#6755=VERTEX_POINT ( 'NONE', #8538 ) ;
#6763=DIRECTION ( 'NONE',  ( -0.000000000000000000, 1.000000000000000000, -0.000000000000000000 ) ) ;
#6772=CARTESIAN_POINT ( 'NONE',  ( -4.458734125000000326, -22.00000000136559208, -1.846868145590735644 ) ) ;
#6775=FACE_OUTER_BOUND ( 'NONE', #8649, .T. ) ;
#6778=CARTESIAN_POINT ( 'NONE',  ( 1.846868145590736310, -22.62500000136559564, 4.458734124999999437 ) ) ;
#6786=CARTESIAN_POINT ( 'NONE',  ( -5.000000000000000000, -24.50000000000000000, -6.123233995736766282E-16 ) ) ;
#6790=CARTESIAN_POINT ( 'NONE',  ( -3.535533905932737309, -23.75000000273118772, -3.535533905932738197 ) ) ;
#6792=CARTESIAN_POINT ( 'NONE',  ( 4.458734124999999437, -28.37500000136559564, -1.846868145590734978 ) ) ;
#6799=DIRECTION ( 'NONE',  ( 0.000000000000000000, 0.000000000000000000, 1.000000000000000000 ) ) ;
#6801=CARTESIAN_POINT ( 'NONE',  ( -9.184850993605147944E-16, -24.37500000273118772, 5.000000000000000000 ) ) ;
#6806=CARTESIAN_POINT ( 'NONE',  ( 1.846868145590735200, -29.50000000136559564, -4.458734125000000326 ) ) ;
#6825=( NAMED_UNIT ( * ) SI_UNIT ( $, .STERADIAN. ) SOLID_ANGLE_UNIT ( ) );
#6839=CYLINDRICAL_SURFACE ( 'NONE', #12798, 5.000000000000000000 ) ;
#6840=EDGE_CURVE ( 'NONE', #13973, #3228, #503, .T. ) ;
#6850=CARTESIAN_POINT ( 'NONE',  ( 3.152801135295367541, -28.56250000136559564, -3.152801135295367541 ) ) ;
#6860=CARTESIAN_POINT ( 'NONE',  ( -4.458734125000000326, -25.25000000136559564, -1.846868145590735644 ) ) ;
#6868=CARTESIAN_POINT ( 'NONE',  ( -3.535533905932737309, -24.62500000000000000, -3.535533905932738197 ) ) ;
#6873=CARTESIAN_POINT ( 'NONE',  ( -5.000000000000000888, -21.68750000273119127, -2.071067811865475949 ) ) ;
#6877=CARTESIAN_POINT ( 'NONE',  ( 2.730187237215162345E-16, -27.18750000136559564, -4.458734124999999437 ) ) ;
#6884=( BOUNDED_CURVE ( )  B_SPLINE_CURVE ( 2, ( #7122, #12024, #8185, #1937, #15609, #898, #818, #973, #6801 ),
 .UNSPECIFIED., .F., .F. ) 
 B_SPLINE_CURVE_WITH_KNOTS ( ( 3, 2, 2, 2, 3 ),
 ( 0.6250000000000002220, 0.6375000000000000666, 0.6500000000000001332, 0.6624999999999999778, 0.6749999999999999334 ),
 .UNSPECIFIED. ) 
 CURVE ( )  GEOMETRIC_REPRESENTATION_ITEM ( )  RATIONAL_B_SPLINE_CURVE ( ( 0.9999999999999986677, 0.9238795325112880708, 1.000000000000000000, 0.9238795325112867385, 1.000000000000000000, 0.9238795325112867385, 1.000000000000000000, 0.9238795325112874046, 0.9999999999999993339 ) ) 
 REPRESENTATION_ITEM ( '' )  );
#6885=AXIS2_PLACEMENT_3D ( 'NONE', #9584, #13279, #2144 ) ;
#6890=CARTESIAN_POINT ( 'NONE',  ( 4.458734125000000326, -26.62500000136559564, -1.846868145590734978 ) ) ;
#6896=ADVANCED_FACE ( 'NONE', ( #10221, #6669 ), #15149, .F. ) ;
#6898=EDGE_CURVE ( 'NONE', #13770, #10095, #5131, .T. ) ;
#6912=CARTESIAN_POINT ( 'NONE',  ( 5.000000000000000888, -24.93750000000000355, -2.071067811865475505 ) ) ;
#6919=CARTESIAN_POINT ( 'NONE',  ( 2.071067811865491048, -27.18750000000000000, 4.999999999999985789 ) ) ;
#6922=ORIENTED_EDGE ( 'NONE', *, *, #446, .T. ) ;
#6924=CARTESIAN_POINT ( 'NONE',  ( 3.061616997868383141E-16, -29.87500000273118417, -5.000000000000000000 ) ) ;
#6929=DIRECTION ( 'NONE',  ( 0.000000000000000000, 0.000000000000000000, 1.000000000000000000 ) ) ;
#6935=EDGE_CURVE ( 'NONE', #10196, #2292, #4788, .T. ) ;
#6936=CARTESIAN_POINT ( 'NONE',  ( 1.846868145590735200, -31.50000000136559564, -4.458734124999999437 ) ) ;
#6938=EDGE_CURVE ( 'NONE', #5212, #15819, #3980, .T. ) ;
#6942=VECTOR ( 'NONE', #8856, 1000.000000000000000 ) ;
#6944=ORIENTED_EDGE ( 'NONE', *, *, #15306, .F. ) ;
#6947=CARTESIAN_POINT ( 'NONE',  ( 3.152801135295367541, -26.56250000136559564, -3.152801135295367541 ) ) ;
#6956=CARTESIAN_POINT ( 'NONE',  ( -3.535533905932738641, -27.37500000000000000, 3.535533905932737309 ) ) ;
#6960=CARTESIAN_POINT ( 'NONE',  ( -3.152801135295367096, -30.06250000136559564, -3.152801135295367541 ) ) ;
#6968=CARTESIAN_POINT ( 'NONE',  ( -1.846868145590737420, -27.75000000136559564, 4.458734124999999437 ) ) ;
#6974=CARTESIAN_POINT ( 'NONE',  ( 2.730187237215162345E-16, -26.43750000136559564, -4.458734124999999437 ) ) ;
#6977=CARTESIAN_POINT ( 'NONE',  ( 2.071067811865461294, -30.81249999999999645, -5.000000000000014211 ) ) ;
#6987=EDGE_CURVE ( 'NONE', #11826, #4598, #7986, .T. ) ;
#6993=CARTESIAN_POINT ( 'NONE',  ( 3.061616997868383043E-15, 20.00000000000000000, -25.00000000000000000 ) ) ;
#7000=ORIENTED_EDGE ( 'NONE', *, *, #499, .F. ) ;
#7013=CARTESIAN_POINT ( 'NONE',  ( 4.458734124999997661, -28.75000000136559564, 1.846868145590737864 ) ) ;
#7015=ORIENTED_EDGE ( 'NONE', *, *, #14503, .T. ) ;
#7021=CARTESIAN_POINT ( 'NONE',  ( -4.458734125000001214, -28.12500000136559564, 1.846868145590734089 ) ) ;
#7033=CARTESIAN_POINT ( 'NONE',  ( 4.458734124999999437, -30.43750000136559564, 0.000000000000000000 ) ) ;
#7035=CARTESIAN_POINT ( 'NONE',  ( 3.152801135295367541, -23.31250000136559564, -3.152801135295367541 ) ) ;
#7040=CARTESIAN_POINT ( 'NONE',  ( 1.846868145590735200, -30.25000000136559564, -4.458734125000000326 ) ) ;
#7047=CARTESIAN_POINT ( 'NONE',  ( -4.458734125000000326, -26.25000000136559208, -1.846868145590735644 ) ) ;
#7050=CARTESIAN_POINT ( 'NONE',  ( 3.061616997868383141E-16, -30.87500000273118772, -5.000000000000000000 ) ) ;
#7063=ORIENTED_EDGE ( 'NONE', *, *, #13884, .F. ) ;
#7072=EDGE_LOOP ( 'NONE', ( #11633, #7367, #1480, #14513 ) ) ;
#7079=ORIENTED_EDGE ( 'NONE', *, *, #14466, .F. ) ;
#7087=CARTESIAN_POINT ( 'NONE',  ( 0.000000000000000000, -11.00000000000000178, 0.000000000000000000 ) ) ;
#7088=CARTESIAN_POINT ( 'NONE',  ( 4.458734124999999437, -31.68750000136559564, 0.000000000000000000 ) ) ;
#7094=ORIENTED_EDGE ( 'NONE', *, *, #4507, .T. ) ;
#7099=CARTESIAN_POINT ( 'NONE',  ( 2.730187237215162345E-16, -28.43750000136559564, -4.458734124999999437 ) ) ;
#7106=CARTESIAN_POINT ( 'NONE',  ( -5.000000000000000888, -22.56250000000000000, -2.071067811865475949 ) ) ;
#7110=CARTESIAN_POINT ( 'NONE',  ( 2.071067811865476394, -22.31250000273118417, 5.000000000000000000 ) ) ;
#7117=EDGE_CURVE ( 'NONE', #13476, #4620, #2415, .T. ) ;
#7119=CARTESIAN_POINT ( 'NONE',  ( -3.152801135295367985, -29.81250000136559208, 3.152801135295367096 ) ) ;
#7122=CARTESIAN_POINT ( 'NONE',  ( 3.061616997868383141E-16, -24.87500000273118417, -4.999999999999999112 ) ) ;
#7128=CARTESIAN_POINT ( 'NONE',  ( 4.458734124999999437, -24.68750000136559564, 0.000000000000000000 ) ) ;
#7142=CARTESIAN_POINT ( 'NONE',  ( 3.061616997868383141E-16, -26.75000000000000000, -5.000000000000000000 ) ) ;
#7158=ORIENTED_EDGE ( 'NONE', *, *, #8592, .T. ) ;
#7161=EDGE_LOOP ( 'NONE', ( #11373, #10810, #5922, #813 ) ) ;
#7162=AXIS2_PLACEMENT_3D ( 'NONE', #10363, #9077, #11325 ) ;
#7164=ADVANCED_FACE ( 'NONE', ( #1139 ), #3482, .F. ) ;
#7166=VECTOR ( 'NONE', #11676, 1000.000000000000000 ) ;
#7172=CARTESIAN_POINT ( 'NONE',  ( 4.458734124999997661, -30.75000000136559919, 1.846868145590737864 ) ) ;
#7174=ORIENTED_EDGE ( 'NONE', *, *, #8975, .T. ) ;
#7181=CARTESIAN_POINT ( 'NONE',  ( 4.458734124999999437, -25.75000000136559564, 1.846868145590737864 ) ) ;
#7195=CARTESIAN_POINT ( 'NONE',  ( 3.152801135295366208, -30.56250000136559564, 3.152801135295367985 ) ) ;
#7203=CARTESIAN_POINT ( 'NONE',  ( -1.846868145590734756, -29.12500000136559919, -4.458734125000000326 ) ) ;
#7207=VECTOR ( 'NONE', #257, 1000.000000000000000 ) ;
#7212=CARTESIAN_POINT ( 'NONE',  ( 3.152801135295367541, -22.56250000136559564, -3.152801135295367541 ) ) ;
#7214=CARTESIAN_POINT ( 'NONE',  ( -9.184850993605147944E-16, -28.37500000273118772, 5.000000000000000000 ) ) ;
#7221=ORIENTED_EDGE ( 'NONE', *, *, #9727, .F. ) ;
#7222=CYLINDRICAL_SURFACE ( 'NONE', #414, 5.999999999999991118 ) ;
#7237=PRESENTATION_STYLE_ASSIGNMENT (( #13346 ) ) ;
#7243=ADVANCED_FACE ( 'NONE', ( #5436, #2670 ), #352, .F. ) ;
#7250=CARTESIAN_POINT ( 'NONE',  ( -9.184850993605147944E-16, -22.37500000273118417, 5.000000000000000000 ) ) ;
#7251=CARTESIAN_POINT ( 'NONE',  ( 2.730187237215162345E-16, -26.43750000136559564, -4.458734124999999437 ) ) ;
#7253=DIRECTION ( 'NONE',  ( 0.000000000000000000, 1.000000000000000000, 0.000000000000000000 ) ) ;
#7258=CARTESIAN_POINT ( 'NONE',  ( -3.152801135295367096, -24.31250000136559564, -3.152801135295367541 ) ) ;
#7259=CARTESIAN_POINT ( 'NONE',  ( 6.123233995736766282E-16, -32.00000000000000000, -5.000000000000000000 ) ) ;
#7267=CARTESIAN_POINT ( 'NONE',  ( -4.458734125000000326, -28.00000000136559564, -1.846868145590735644 ) ) ;
#7272=VERTEX_POINT ( 'NONE', #8833 ) ;
#7274=CARTESIAN_POINT ( 'NONE',  ( -1.846868145590734756, -24.12500000136559919, -4.458734125000000326 ) ) ;
#7275=EDGE_CURVE ( 'NONE', #2433, #11572, #2756, .T. ) ;
#7282=CARTESIAN_POINT ( 'NONE',  ( 4.458734125000000326, -22.62500000136559564, -1.846868145590734978 ) ) ;
#7285=CARTESIAN_POINT ( 'NONE',  ( 3.535533905932738197, -30.87500000000000000, -3.535533905932738197 ) ) ;
#7291=ADVANCED_FACE ( 'NONE', ( #3889 ), #2941, .T. ) ;
#7293=DIRECTION ( 'NONE',  ( 0.000000000000000000, 0.000000000000000000, -1.000000000000000000 ) ) ;
#7300=CARTESIAN_POINT ( 'NONE',  ( 2.071067811865468844, -27.81250000000000000, -5.000000000000007994 ) ) ;
#7306=FILL_AREA_STYLE_COLOUR ( '', #10238 ) ;
#7317=DIRECTION ( 'NONE',  ( -0.000000000000000000, 1.000000000000000000, -0.000000000000000000 ) ) ;
#7322=CARTESIAN_POINT ( 'NONE',  ( -8.190561711645485556E-16, -24.93750000136559564, 4.458734124999999437 ) ) ;
#7323=CARTESIAN_POINT ( 'NONE',  ( 2.730187237215162345E-16, -23.18750000136559564, -4.458734124999999437 ) ) ;
#7332=DIRECTION ( 'NONE',  ( -8.881784197001252323E-15, 0.000000000000000000, 1.000000000000000000 ) ) ;
#7337=CARTESIAN_POINT ( 'NONE',  ( -3.535533905932737309, -23.62500000000000000, -3.535533905932738197 ) ) ;
#7339=DIRECTION ( 'NONE',  ( 0.000000000000000000, -1.000000000000000000, 0.000000000000000000 ) ) ;
#7341=CARTESIAN_POINT ( 'NONE',  ( 2.730187237215162345E-16, -28.18750000136559564, -4.458734124999999437 ) ) ;
#7350=CARTESIAN_POINT ( 'NONE',  ( 3.152801135295366208, -25.56250000136559564, 3.152801135295367985 ) ) ;
#7354=LINE ( 'NONE', #10985, #10480 ) ;
#7358=CARTESIAN_POINT ( 'NONE',  ( -3.152801135295367985, -23.06250000136559564, 3.152801135295367096 ) ) ;
#7359=VECTOR ( 'NONE', #14257, 1000.000000000000000 ) ;
#7362=CARTESIAN_POINT ( 'NONE',  ( 5.000000000000000000, -30.12500000273118417, 0.000000000000000000 ) ) ;
#7367=ORIENTED_EDGE ( 'NONE', *, *, #2620, .T. ) ;
#7371=VERTEX_POINT ( 'NONE', #14530 ) ;
#7391=( BOUNDED_CURVE ( )  B_SPLINE_CURVE ( 2, ( #14746, #15066, #13506, #8616, #10142, #2444, #8778, #9890, #1400 ),
 .UNSPECIFIED., .F., .F. ) 
 B_SPLINE_CURVE_WITH_KNOTS ( ( 3, 2, 2, 2, 3 ),
 ( 0.02500000000000002220, 0.03750000000000003331, 0.05000000000000004441, 0.06250000000000005551, 0.07500000000000006661 ),
 .UNSPECIFIED. ) 
 CURVE ( )  GEOMETRIC_REPRESENTATION_ITEM ( )  RATIONAL_B_SPLINE_CURVE ( ( 0.9999999999999998890, 0.9238795325112868495, 1.000000000000000000, 0.9238795325112867385, 1.000000000000000000, 0.9238795325112867385, 1.000000000000000000, 0.9238795325112862944, 1.000000000000000444 ) ) 
 REPRESENTATION_ITEM ( '' )  );
#7395=AXIS2_PLACEMENT_3D ( 'NONE', #401, #5169, #14953 ) ;
#7397=DIRECTION ( 'NONE',  ( 0.000000000000000000, 1.000000000000000000, 0.000000000000000000 ) ) ;
#7405=CARTESIAN_POINT ( 'NONE',  ( -4.458734124999999437, -27.25000000136559564, -1.846868145590735644 ) ) ;
#7406=CARTESIAN_POINT ( 'NONE',  ( 3.152801135295367541, -24.31250000136559564, -3.152801135295367541 ) ) ;
#7409=ORIENTED_EDGE ( 'NONE', *, *, #15324, .F. ) ;
#7415=CARTESIAN_POINT ( 'NONE',  ( 3.152801135295366208, -23.81250000136559564, 3.152801135295367985 ) ) ;
#7417=CARTESIAN_POINT ( 'NONE',  ( 5.000000000000000888, -30.06250000273118417, -2.071067811865475505 ) ) ;
#7428=CARTESIAN_POINT ( 'NONE',  ( -1.846868145590737420, -26.75000000136559564, 4.458734124999999437 ) ) ;
#7437=CARTESIAN_POINT ( 'NONE',  ( -3.152801135295367985, -22.81250000136559564, 3.152801135295367096 ) ) ;
#7438=CARTESIAN_POINT ( 'NONE',  ( 6.123233995736766282E-16, -20.00000000000000000, -5.000000000000000000 ) ) ;
#7439=ORIENTED_EDGE ( 'NONE', *, *, #15652, .T. ) ;
#7440=AXIS2_PLACEMENT_3D ( 'NONE', #12633, #9100, #1576 ) ;
#7447=CARTESIAN_POINT ( 'NONE',  ( 3.152801135295367541, -24.56250000136559564, -3.152801135295367541 ) ) ;
#7451=CARTESIAN_POINT ( 'NONE',  ( 3.535533905932738197, -30.00000000273118417, -3.535533905932738197 ) ) ;
#7452=CARTESIAN_POINT ( 'NONE',  ( -9.184850993605147944E-16, -29.37500000273118417, 5.000000000000000000 ) ) ;
#7454=CARTESIAN_POINT ( 'NONE',  ( 4.458734124999999437, -29.37500000136559208, -1.846868145590734978 ) ) ;
#7462=AXIS2_PLACEMENT_3D ( 'NONE', #2501, #3649, #13334 ) ;
#7471=DIRECTION ( 'NONE',  ( 0.000000000000000000, 0.000000000000000000, 1.000000000000000000 ) ) ;
#7474=CYLINDRICAL_SURFACE ( 'NONE', #949, 6.000000000000000888 ) ;
#7475=ORIENTED_EDGE ( 'NONE', *, *, #3327, .F. ) ;
#7478=EDGE_CURVE ( 'NONE', #11064, #2143, #12648, .T. ) ;
#7481=DIRECTION ( 'NONE',  ( 1.000000000000000000, 0.000000000000000000, 0.000000000000000000 ) ) ;
#7482=DIRECTION ( 'NONE',  ( 0.000000000000000000, 0.000000000000000000, 1.000000000000000000 ) ) ;
#7487=CARTESIAN_POINT ( 'NONE',  ( 4.458734124999999437, -27.62500000136559564, -1.846868145590734978 ) ) ;
#7489=CARTESIAN_POINT ( 'NONE',  ( -1.846868145590737420, -22.75000000136559919, 4.458734124999997661 ) ) ;
#7494=( BOUNDED_CURVE ( )  B_SPLINE_CURVE ( 2, ( #6591, #6683, #3026, #5535, #10470, #11505, #376, #14013, #9182 ),
 .UNSPECIFIED., .F., .F. ) 
 B_SPLINE_CURVE_WITH_KNOTS ( ( 3, 2, 2, 2, 3 ),
 ( 0.4250000000000000444, 0.4375000000000000555, 0.4500000000000000666, 0.4625000000000001332, 0.4750000000000000888 ),
 .UNSPECIFIED. ) 
 CURVE ( )  GEOMETRIC_REPRESENTATION_ITEM ( )  RATIONAL_B_SPLINE_CURVE ( ( 0.9999999999999996669, 0.9238795325112870716, 1.000000000000000000, 0.9238795325112867385, 1.000000000000000000, 0.9238795325112867385, 1.000000000000000000, 0.9238795325112860723, 1.000000000000000666 ) ) 
 REPRESENTATION_ITEM ( '' )  );
#7495=SHAPE_REPRESENTATION ( 'Drive Unit', ( #3223 ), #15660 ) ;
#7498=CARTESIAN_POINT ( 'NONE',  ( 5.000000000000000888, -31.06250000273118772, -2.071067811865475505 ) ) ;
#7500=CARTESIAN_POINT ( 'NONE',  ( 4.458734124999999437, -21.56250000136559208, 0.000000000000000000 ) ) ;
#7509=CARTESIAN_POINT ( 'NONE',  ( 4.458734124999999437, -27.43750000136559564, 0.000000000000000000 ) ) ;
#7512=DIRECTION ( 'NONE',  ( 0.000000000000000000, 1.000000000000000000, 0.000000000000000000 ) ) ;
#7516=CARTESIAN_POINT ( 'NONE',  ( 2.730187237215162345E-16, -25.18750000136559564, -4.458734124999999437 ) ) ;
#7525=CARTESIAN_POINT ( 'NONE',  ( 2.071067811865476394, -30.18750000000000711, 5.000000000000000000 ) ) ;
#7527=LINE ( 'NONE', #4194, #14912 ) ;
#7528=CARTESIAN_POINT ( 'NONE',  ( -5.000000000000000888, -26.56250000273118417, 2.071067811865474617 ) ) ;
#7531=CARTESIAN_POINT ( 'NONE',  ( 4.458734124999999437, -29.43750000136559208, 0.000000000000000000 ) ) ;
#7533=ORIENTED_EDGE ( 'NONE', *, *, #15514, .T. ) ;
#7549=CARTESIAN_POINT ( 'NONE',  ( 3.061616997868383141E-16, -23.75000000000000000, -5.000000000000000000 ) ) ;
#7562=DIRECTION ( 'NONE',  ( 0.000000000000000000, -1.000000000000000000, 0.000000000000000000 ) ) ;
#7568=CARTESIAN_POINT ( 'NONE',  ( 3.535533905932736864, -28.25000000273118772, 3.535533905932738641 ) ) ;
#7569=CARTESIAN_POINT ( 'NONE',  ( -3.152801135295367096, -25.31250000136559564, -3.152801135295367541 ) ) ;
#7575=ORIENTED_EDGE ( 'NONE', *, *, #1179, .T. ) ;
#7576=ORIENTED_EDGE ( 'NONE', *, *, #6987, .T. ) ;
#7578=CARTESIAN_POINT ( 'NONE',  ( 3.152801135295366208, -21.81250000136559208, 3.152801135295367985 ) ) ;
#7579=CARTESIAN_POINT ( 'NONE',  ( 0.000000000000000000, -20.00000000000000000, 0.000000000000000000 ) ) ;
#7587=CARTESIAN_POINT ( 'NONE',  ( 3.061616997868383141E-16, -28.75000000000000000, -5.000000000000000000 ) ) ;
#7589=CARTESIAN_POINT ( 'NONE',  ( -3.152801135295367096, -28.06250000136559564, -3.152801135295367541 ) ) ;
#7594=EDGE_LOOP ( 'NONE', ( #4407, #12194, #10051 ) ) ;
#7596=CARTESIAN_POINT ( 'NONE',  ( 3.152801135295367541, -24.31250000136559564, -3.152801135295367541 ) ) ;
#7603=DIRECTION ( 'NONE',  ( -0.000000000000000000, 1.000000000000000000, -0.000000000000000000 ) ) ;
#7604=CARTESIAN_POINT ( 'NONE',  ( -9.184850993605147944E-16, -29.25000000000000000, 5.000000000000000000 ) ) ;
#7606=CARTESIAN_POINT ( 'NONE',  ( -35.00000000000000000, 37.00000000000000000, -2.649999999999985700 ) ) ;
#7607=ADVANCED_FACE ( 'NONE', ( #12724 ), #13945, .T. ) ;
#7608=CARTESIAN_POINT ( 'NONE',  ( 5.000000000000000888, -30.06250000273118417, -2.071067811865475505 ) ) ;
#7611=CARTESIAN_POINT ( 'NONE',  ( -1.846868145590737420, -29.75000000136559564, 4.458734124999997661 ) ) ;
#7614=ORIENTED_EDGE ( 'NONE', *, *, #12797, .F. ) ;
#7616=ORIENTED_EDGE ( 'NONE', *, *, #8377, .F. ) ;
#7621=CARTESIAN_POINT ( 'NONE',  ( -9.184850993605147944E-16, -31.25000000000000000, 5.000000000000000000 ) ) ;
#7623=CARTESIAN_POINT ( 'NONE',  ( 0.000000000000000000, -20.00000000000000000, 5.000000000000000000 ) ) ;
#7631=CARTESIAN_POINT ( 'NONE',  ( 35.00000000000000000, 37.00000000000000000, -5.999999999999991118 ) ) ;
#7633=ORIENTED_EDGE ( 'NONE', *, *, #4427, .F. ) ;
#7645=DIRECTION ( 'NONE',  ( -0.000000000000000000, 1.000000000000000000, -0.000000000000000000 ) ) ;
#7648=ADVANCED_FACE ( 'NONE', ( #469 ), #7989, .F. ) ;
#7660=ORIENTED_EDGE ( 'NONE', *, *, #10590, .F. ) ;
#7665=CARTESIAN_POINT ( 'NONE',  ( 3.061616997868383141E-16, -25.75000000000000355, -5.000000000000000000 ) ) ;
#7667=AXIS2_PLACEMENT_3D ( 'NONE', #432, #356, #6494 ) ;
#7674=CARTESIAN_POINT ( 'NONE',  ( 1.846868145590735200, -22.25000000136559564, -4.458734125000000326 ) ) ;
#7680=CARTESIAN_POINT ( 'NONE',  ( 2.730187237215162345E-16, -30.43750000136559564, -4.458734124999999437 ) ) ;
#7692=CARTESIAN_POINT ( 'NONE',  ( 3.535533905932736864, -28.12500000000000000, 3.535533905932738641 ) ) ;
#7696=CARTESIAN_POINT ( 'NONE',  ( 5.000000000000000000, -27.12500000273118772, 0.000000000000000000 ) ) ;
#7698=CARTESIAN_POINT ( 'NONE',  ( 2.071067811865462183, -24.31250000273118417, 5.000000000000013323 ) ) ;
#7706=DIRECTION ( 'NONE',  ( -0.000000000000000000, 1.000000000000000000, -0.000000000000000000 ) ) ;
#7711=CARTESIAN_POINT ( 'NONE',  ( -2.071067811865469288, -31.31250000000000000, 5.000000000000007994 ) ) ;
#7712=CARTESIAN_POINT ( 'NONE',  ( -4.458734125000000326, -31.25000000136559564, -1.846868145590735644 ) ) ;
#7720=STYLED_ITEM ( 'NONE', ( #7810 ), #9346 ) ;
#7729=EDGE_CURVE ( 'NONE', #11572, #10095, #11809, .T. ) ;
#7734=CARTESIAN_POINT ( 'NONE',  ( 5.000000000000000000, -21.12500000273118772, 0.000000000000000000 ) ) ;
#7740=DIRECTION ( 'NONE',  ( 0.000000000000000000, 0.000000000000000000, -1.000000000000000000 ) ) ;
#7744=LINE ( 'NONE', #15161, #6360 ) ;
#7745=ORIENTED_EDGE ( 'NONE', *, *, #1953, .T. ) ;
#7759=CARTESIAN_POINT ( 'NONE',  ( 3.535533905932736864, -30.12500000000000000, 3.535533905932738641 ) ) ;
#7760=CARTESIAN_POINT ( 'NONE',  ( 5.000000000000000000, -29.00000000000000000, 0.000000000000000000 ) ) ;
#7761=CARTESIAN_POINT ( 'NONE',  ( 3.152801135295367541, -23.31250000136559564, -3.152801135295367541 ) ) ;
#7765=ORIENTED_EDGE ( 'NONE', *, *, #6938, .F. ) ;
#7768=CARTESIAN_POINT ( 'NONE',  ( -1.846868145590737420, -22.75000000136559208, 4.458734124999999437 ) ) ;
#7771=CARTESIAN_POINT ( 'NONE',  ( -2.071067811865468400, -28.68750000000000000, -5.000000000000007994 ) ) ;
#7775=CARTESIAN_POINT ( 'NONE',  ( 3.535533905932738197, -31.87500000000000000, -3.535533905932738197 ) ) ;
#7778=CARTESIAN_POINT ( 'NONE',  ( -5.000000000000000000, -22.62500000273118772, -6.123233995736766282E-16 ) ) ;
#7780=CARTESIAN_POINT ( 'NONE',  ( -4.458734124999999437, -26.00000000136559564, -1.846868145590735644 ) ) ;
#7781=EDGE_CURVE ( 'NONE', #6661, #10619, #6023, .T. ) ;
#7782=DIRECTION ( 'NONE',  ( 0.000000000000000000, 0.000000000000000000, 1.000000000000000000 ) ) ;
#7783=ORIENTED_EDGE ( 'NONE', *, *, #9727, .T. ) ;
#7789=CARTESIAN_POINT ( 'NONE',  ( 1.846868145590736310, -29.87500000136559564, 4.458734124999999437 ) ) ;
#7794=EDGE_CURVE ( 'NONE', #4537, #15165, #4094, .T. ) ;
#7796=EDGE_CURVE ( 'NONE', #12412, #580, #4604, .T. ) ;
#7798=EDGE_LOOP ( 'NONE', ( #14156, #529, #308, #3677 ) ) ;
#7800=CARTESIAN_POINT ( 'NONE',  ( -4.458734125000001214, -30.87500000136559564, 1.846868145590734089 ) ) ;
#7801=ORIENTED_EDGE ( 'NONE', *, *, #10465, .F. ) ;
#7807=CARTESIAN_POINT ( 'NONE',  ( 2.071067811865476394, -28.18750000000000355, 5.000000000000000000 ) ) ;
#7810=PRESENTATION_STYLE_ASSIGNMENT (( #9333 ) ) ;
#7811=CARTESIAN_POINT ( 'NONE',  ( -4.458734124999999437, -22.18750000136559564, -5.460374474430324690E-16 ) ) ;
#7812=EDGE_CURVE ( 'NONE', #3489, #11826, #13431, .T. ) ;
#7814=CYLINDRICAL_SURFACE ( 'NONE', #5881, 6.000000000000000888 ) ;
#7819=ORIENTED_EDGE ( 'NONE', *, *, #3701, .F. ) ;
#7821=LINE ( 'NONE', #2869, #11538 ) ;
#7826=CARTESIAN_POINT ( 'NONE',  ( 0.000000000000000000, -13.00000000000000178, 0.000000000000000000 ) ) ;
#7829=CARTESIAN_POINT ( 'NONE',  ( 3.061616997868383141E-16, -29.75000000000000000, -5.000000000000000000 ) ) ;
#7832=CYLINDRICAL_SURFACE ( 'NONE', #15374, 5.000000000000000000 ) ;
#7840=CARTESIAN_POINT ( 'NONE',  ( -4.458734124999999437, -29.18750000136559564, -5.460374474430324690E-16 ) ) ;
#7846=CARTESIAN_POINT ( 'NONE',  ( -2.071067811865475061, -29.68750000000000711, -5.000000000000000888 ) ) ;
#7850=CARTESIAN_POINT ( 'NONE',  ( -5.000000000000000888, -25.68750000273119127, -2.071067811865475949 ) ) ;
#7851=ADVANCED_FACE ( 'NONE', ( #4809 ), #858, .T. ) ;
#7853=CARTESIAN_POINT ( 'NONE',  ( 1.846868145590736310, -26.62500000136559564, 4.458734124999997661 ) ) ;
#7854=DIRECTION ( 'NONE',  ( 0.000000000000000000, 1.000000000000000000, 0.000000000000000000 ) ) ;
#7863=CARTESIAN_POINT ( 'NONE',  ( -3.535533905932738641, -31.37500000000000000, 3.535533905932737309 ) ) ;
#7864=CARTESIAN_POINT ( 'NONE',  ( 4.458734124999999437, -29.75000000136559564, 1.846868145590737864 ) ) ;
#7867=SHAPE_DEFINITION_REPRESENTATION ( #10928, #7495 ) ;
#7873=CARTESIAN_POINT ( 'NONE',  ( -8.190561711645485556E-16, -27.68750000136559564, 4.458734124999999437 ) ) ;
#7888=ORIENTED_EDGE ( 'NONE', *, *, #6286, .T. ) ;
#7898=CARTESIAN_POINT ( 'NONE',  ( 0.000000000000000000, -20.00000000000000000, 0.000000000000000000 ) ) ;
#7899=CIRCLE ( 'NONE', #6083, 2.649999999999992806 ) ;
#7900=PLANE ( 'NONE',  #9418 ) ;
#7907=CARTESIAN_POINT ( 'NONE',  ( 2.071067811865447528, -24.93750000273118417, -5.000000000000029310 ) ) ;
#7908=CARTESIAN_POINT ( 'NONE',  ( 4.458734124999999437, -24.50000000136559564, 1.846868145590737864 ) ) ;
#7910=EDGE_LOOP ( 'NONE', ( #2022, #12076 ) ) ;
#7915=AXIS2_PLACEMENT_3D ( 'NONE', #1027, #15823, #9660 ) ;
#7916=CARTESIAN_POINT ( 'NONE',  ( 3.152801135295366208, -30.81250000136559564, 3.152801135295367985 ) ) ;
#7918=ORIENTED_EDGE ( 'NONE', *, *, #1483, .T. ) ;
#7929=CARTESIAN_POINT ( 'NONE',  ( -3.535533905932738641, -25.37500000000000000, 3.535533905932737309 ) ) ;
#7934=CARTESIAN_POINT ( 'NONE',  ( -3.535533905932737309, -22.75000000273118772, -3.535533905932738197 ) ) ;
#7936=CARTESIAN_POINT ( 'NONE',  ( -1.846868145590737420, -26.75000000136559564, 4.458734124999997661 ) ) ;
#7938=VERTEX_POINT ( 'NONE', #14826 ) ;
#7946=CARTESIAN_POINT ( 'NONE',  ( 5.809475019311125976, -13.00000000000000178, -1.500000000000000000 ) ) ;
#7949=CARTESIAN_POINT ( 'NONE',  ( -4.458734124999999437, -26.18750000136559919, -5.460374474430324690E-16 ) ) ;
#7954=( NAMED_UNIT ( * ) SI_UNIT ( $, .STERADIAN. ) SOLID_ANGLE_UNIT ( ) );
#7955=CIRCLE ( 'NONE', #15733, 6.000000000000000888 ) ;
#7958=CARTESIAN_POINT ( 'NONE',  ( -8.190561711645485556E-16, -29.68750000136559208, 4.458734124999999437 ) ) ;
#7968=FILL_AREA_STYLE_COLOUR ( '', #12065 ) ;
#7969=CARTESIAN_POINT ( 'NONE',  ( 3.061616997868383141E-16, -28.75000000000000000, -5.000000000000000000 ) ) ;
#7975=ADVANCED_FACE ( 'NONE', ( #12305 ), #1568, .T. ) ;
#7984=DIRECTION ( 'NONE',  ( 0.000000000000000000, -0.000000000000000000, 1.000000000000000000 ) ) ;
#7986=CIRCLE ( 'NONE', #1512, 6.000000000000000888 ) ;
#7987=DIRECTION ( 'NONE',  ( -0.000000000000000000, 1.000000000000000000, -0.000000000000000000 ) ) ;
#7989=PLANE ( 'NONE',  #12347 ) ;
#7994=CARTESIAN_POINT ( 'NONE',  ( 2.730187237215162345E-16, -24.18750000136559564, -4.458734124999999437 ) ) ;
#7995=AXIS2_PLACEMENT_3D ( 'NONE', #9767, #13541, #13457 ) ;
#7999=EDGE_CURVE ( 'NONE', #15267, #8315, #7391, .T. ) ;
#8000=ORIENTED_EDGE ( 'NONE', *, *, #11671, .F. ) ;
#8004=CARTESIAN_POINT ( 'NONE',  ( 2.730187237215162345E-16, -29.43750000136559208, -4.458734124999999437 ) ) ;
#8012=CARTESIAN_POINT ( 'NONE',  ( 3.061616997868383141E-16, -24.75000000000000000, -5.000000000000000000 ) ) ;
#8016=CARTESIAN_POINT ( 'NONE',  ( 3.535533905932736864, -24.25000000273118772, 3.535533905932738641 ) ) ;
#8018=CARTESIAN_POINT ( 'NONE',  ( 1.846868145590736310, -25.62500000136559564, 4.458734124999997661 ) ) ;
#8019=EDGE_CURVE ( 'NONE', #6755, #3455, #13447, .T. ) ;
#8022=ORIENTED_EDGE ( 'NONE', *, *, #4689, .F. ) ;
#8028=( BOUNDED_CURVE ( )  B_SPLINE_CURVE ( 2, ( #5782, #11035, #2305, #13364, #4729, #9735, #4653, #13510, #7250 ),
 .UNSPECIFIED., .F., .F. ) 
 B_SPLINE_CURVE_WITH_KNOTS ( ( 3, 2, 2, 2, 3 ),
 ( 0.8250000000000000666, 0.8375000000000001332, 0.8500000000000000888, 0.8625000000000000444, 0.8750000000000000000 ),
 .UNSPECIFIED. ) 
 CURVE ( )  GEOMETRIC_REPRESENTATION_ITEM ( )  RATIONAL_B_SPLINE_CURVE ( ( 0.9999999999999993339, 0.9238795325112874046, 1.000000000000000000, 0.9238795325112867385, 1.000000000000000000, 0.9238795325112867385, 1.000000000000000000, 0.9238795325112867385, 1.000000000000000000 ) ) 
 REPRESENTATION_ITEM ( '' )  );
#8032=CARTESIAN_POINT ( 'NONE',  ( -1.846868145590737420, -27.00000000136559208, 4.458734124999999437 ) ) ;
#8039=ORIENTED_EDGE ( 'NONE', *, *, #250, .F. ) ;
#8045=DIRECTION ( 'NONE',  ( 0.000000000000000000, 1.000000000000000000, 0.000000000000000000 ) ) ;
#8067=CARTESIAN_POINT ( 'NONE',  ( -5.000000000000000888, -25.56250000000000355, -2.071067811865475949 ) ) ;
#8068=CARTESIAN_POINT ( 'NONE',  ( -9.184850993605147944E-16, -23.25000000000000000, 5.000000000000000000 ) ) ;
#8071=AXIS2_PLACEMENT_3D ( 'NONE', #2029, #15613, #4533 ) ;
#8072=CARTESIAN_POINT ( 'NONE',  ( 5.000000000000000000, -25.18750000273118772, 2.071067811865478614 ) ) ;
#8073=CARTESIAN_POINT ( 'NONE',  ( -4.458734124999999437, -29.18750000136559564, -5.460374474430324690E-16 ) ) ;
#8077=DIRECTION ( 'NONE',  ( 0.000000000000000000, 1.000000000000000000, 0.000000000000000000 ) ) ;
#8078=ORIENTED_EDGE ( 'NONE', *, *, #11102, .F. ) ;
#8081=CARTESIAN_POINT ( 'NONE',  ( -4.458734124999999437, -25.18750000136559564, -5.460374474430324690E-16 ) ) ;
#8085=EDGE_CURVE ( 'NONE', #12657, #379, #11953, .T. ) ;
#8090=CARTESIAN_POINT ( 'NONE',  ( 2.071067811865476394, -27.18750000000000355, 5.000000000000000000 ) ) ;
#8094=CARTESIAN_POINT ( 'NONE',  ( 5.000000000000000000, -24.18750000273119127, 2.071067811865478614 ) ) ;
#8096=CARTESIAN_POINT ( 'NONE',  ( -8.190561711645485556E-16, -25.68750000136559564, 4.458734124999999437 ) ) ;
#8109=CARTESIAN_POINT ( 'NONE',  ( 4.458734124999999437, -25.68750000136559564, 0.000000000000000000 ) ) ;
#8111=CARTESIAN_POINT ( 'NONE',  ( 4.729367062499999719, -31.84375000068279959, 0.000000000000000000 ) ) ;
#8115=( BOUNDED_CURVE ( )  B_SPLINE_CURVE ( 2, ( #9520, #14452, #13375, #12159, #1174, #6120, #5858, #14521, #11047 ),
 .UNSPECIFIED., .F., .F. ) 
 B_SPLINE_CURVE_WITH_KNOTS ( ( 3, 2, 2, 2, 3 ),
 ( 0.7249999999999999778, 0.7375000000000000444, 0.7500000000000000000, 0.7624999999999999556, 0.7750000000000000222 ),
 .UNSPECIFIED. ) 
 CURVE ( )  GEOMETRIC_REPRESENTATION_ITEM ( )  RATIONAL_B_SPLINE_CURVE ( ( 1.000000000000000000, 0.9238795325112867385, 1.000000000000000000, 0.9238795325112867385, 1.000000000000000000, 0.9238795325112867385, 1.000000000000000000, 0.9238795325112867385, 1.000000000000000000 ) ) 
 REPRESENTATION_ITEM ( '' )  );
#8127=LINE ( 'NONE', #5847, #13729 ) ;
#8129=CARTESIAN_POINT ( 'NONE',  ( -9.184850993605147944E-16, -25.25000000000000000, 5.000000000000000000 ) ) ;
#8134=ORIENTED_EDGE ( 'NONE', *, *, #12125, .T. ) ;
#8138=VERTEX_POINT ( 'NONE', #10442 ) ;
#8142=EDGE_CURVE ( 'NONE', #9203, #10564, #5746, .T. ) ;
#8150=CARTESIAN_POINT ( 'NONE',  ( -9.184850993605147944E-16, -25.37500000273118417, 4.999999999999999112 ) ) ;
#8151=CARTESIAN_POINT ( 'NONE',  ( -3.152801135295367985, -28.06250000136559564, 3.152801135295367096 ) ) ;
#8158=CARTESIAN_POINT ( 'NONE',  ( -4.458734125000000326, -27.25000000136559564, -1.846868145590735644 ) ) ;
#8166=CARTESIAN_POINT ( 'NONE',  ( -2.071067811865478170, -27.31250000000000000, 5.000000000000000000 ) ) ;
#8171=CARTESIAN_POINT ( 'NONE',  ( -1.846868145590734756, -29.12500000136559919, -4.458734125000000326 ) ) ;
#8175=CARTESIAN_POINT ( 'NONE',  ( -3.152801135295367096, -22.06250000136559564, -3.152801135295367541 ) ) ;
#8184=ORIENTED_EDGE ( 'NONE', *, *, #8832, .T. ) ;
#8185=CARTESIAN_POINT ( 'NONE',  ( -3.535533905932737309, -24.75000000273118417, -3.535533905932738197 ) ) ;
#8188=CARTESIAN_POINT ( 'NONE',  ( -4.458734125000000326, -27.25000000136559564, -1.846868145590735644 ) ) ;
#8198=ORIENTED_EDGE ( 'NONE', *, *, #12086, .T. ) ;
#8203=LINE ( 'NONE', #12776, #13272 ) ;
#8217=VERTEX_POINT ( 'NONE', #13403 ) ;
#8219=EDGE_LOOP ( 'NONE', ( #6638, #5638, #4955, #2727, #7221, #12338 ) ) ;
#8223=AXIS2_PLACEMENT_3D ( 'NONE', #15568, #6763, #1817 ) ;
#8232=DIRECTION ( 'NONE',  ( 0.000000000000000000, 0.000000000000000000, 1.000000000000000000 ) ) ;
#8235=CARTESIAN_POINT ( 'NONE',  ( -3.152801135295367096, -31.31250000136559564, -3.152801135295367541 ) ) ;
#8241=ORIENTED_EDGE ( 'NONE', *, *, #1440, .T. ) ;
#8243=AXIS2_PLACEMENT_3D ( 'NONE', #1965, #1645, #6753 ) ;
#8247=CARTESIAN_POINT ( 'NONE',  ( -1.846868145590737420, -28.00000000136559564, 4.458734124999999437 ) ) ;
#8250=VECTOR ( 'NONE', #7645, 1000.000000000000000 ) ;
#8255=AXIS2_PLACEMENT_3D ( 'NONE', #8543, #7317, #11033 ) ;
#8257=CARTESIAN_POINT ( 'NONE',  ( -2.071067811865475061, -26.68750000000000355, -5.000000000000000888 ) ) ;
#8261=CARTESIAN_POINT ( 'NONE',  ( 4.458734124999999437, -31.43750000136559564, 0.000000000000000000 ) ) ;
#8263=CARTESIAN_POINT ( 'NONE',  ( 4.458734124999999437, -24.37500000136559564, -1.846868145590734978 ) ) ;
#8264=DIRECTION ( 'NONE',  ( 0.000000000000000000, 1.000000000000000000, 0.000000000000000000 ) ) ;
#8269=CARTESIAN_POINT ( 'NONE',  ( -8.190561711645485556E-16, -30.68750000136559564, 4.458734124999999437 ) ) ;
#8271=EDGE_LOOP ( 'NONE', ( #831, #8184, #909, #3840 ) ) ;
#8276=CARTESIAN_POINT ( 'NONE',  ( 2.730187237215162345E-16, -27.43750000136559564, -4.458734124999999437 ) ) ;
#8279=CARTESIAN_POINT ( 'NONE',  ( 6.123233995736766282E-16, -20.00000000000000000, -5.000000000000000000 ) ) ;
#8280=CARTESIAN_POINT ( 'NONE',  ( 5.000000000000000000, -31.12500000273118772, 0.000000000000000000 ) ) ;
#8295=EDGE_LOOP ( 'NONE', ( #13184, #6482, #10689, #5405, #9683, #5102, #5445, #7000, #3822, #3089, #7614, #4483, #12337, #8022, #11595, #10474, #15381, #15057, #13853, #15731, #3917, #10634, #14009, #8039 ) ) ;
#8313=CARTESIAN_POINT ( 'NONE',  ( -1.846868145590737420, -31.00000000136559564, 4.458734124999997661 ) ) ;
#8315=VERTEX_POINT ( 'NONE', #11547 ) ;
#8320=CARTESIAN_POINT ( 'NONE',  ( 4.458734124999999437, -28.75000000136559208, 1.846868145590737864 ) ) ;
#8321=DIRECTION ( 'NONE',  ( -0.000000000000000000, 1.000000000000000000, -0.000000000000000000 ) ) ;
#8322=FACE_OUTER_BOUND ( 'NONE', #10054, .T. ) ;
#8328=CARTESIAN_POINT ( 'NONE',  ( 5.000000000000000888, -22.93749999999999645, -2.071067811865475505 ) ) ;
#8332=CARTESIAN_POINT ( 'NONE',  ( -1.846868145590737420, -29.75000000136559564, 4.458734124999999437 ) ) ;
#8338=CARTESIAN_POINT ( 'NONE',  ( 4.458734124999999437, -30.50000000136559919, 1.846868145590737864 ) ) ;
#8344=CARTESIAN_POINT ( 'NONE',  ( -3.152801135295367985, -25.06250000136559564, 3.152801135295367096 ) ) ;
#8347=CARTESIAN_POINT ( 'NONE',  ( 3.061616997868383141E-16, -30.75000000000000000, -5.000000000000000000 ) ) ;
#8356=EDGE_LOOP ( 'NONE', ( #13878, #13517, #1073, #10359 ) ) ;
#8364=VECTOR ( 'NONE', #4418, 1000.000000000000000 ) ;
#8365=CARTESIAN_POINT ( 'NONE',  ( 0.000000000000000000, -20.00000000000000000, 5.000000000000000000 ) ) ;
#8368=VERTEX_POINT ( 'NONE', #4117 ) ;
#8371=VERTEX_POINT ( 'NONE', #7606 ) ;
#8374=VERTEX_POINT ( 'NONE', #15203 ) ;
#8377=EDGE_CURVE ( 'NONE', #14100, #15134, #7527, .T. ) ;
#8386=CARTESIAN_POINT ( 'NONE',  ( 4.458734124999999437, -30.62500000136559564, -1.846868145590734978 ) ) ;
#8393=CARTESIAN_POINT ( 'NONE',  ( -3.152801135295367096, -28.31250000136559564, -3.152801135295367541 ) ) ;
#8401=CARTESIAN_POINT ( 'NONE',  ( 2.071067811865475505, -23.81250000000000000, -5.000000000000000888 ) ) ;
#8405=CARTESIAN_POINT ( 'NONE',  ( 2.730187237215162345E-16, -30.18750000136559564, -4.458734124999999437 ) ) ;
#8413=ORIENTED_EDGE ( 'NONE', *, *, #2974, .T. ) ;
#8415=CARTESIAN_POINT ( 'NONE',  ( -3.152801135295367985, -28.81250000136559564, 3.152801135295367096 ) ) ;
#8422=AXIS2_PLACEMENT_3D ( 'NONE', #3314, #8264, #3384 ) ;
#8427=CARTESIAN_POINT ( 'NONE',  ( -8.190561711645485556E-16, -22.93750000136559564, 4.458734124999999437 ) ) ;
#8435=ORIENTED_EDGE ( 'NONE', *, *, #2261, .T. ) ;
#8438=ADVANCED_FACE ( 'NONE', ( #262 ), #5177, .T. ) ;
#8458=DIRECTION ( 'NONE',  ( -1.000000000000000000, 0.000000000000000000, -0.000000000000000000 ) ) ;
#8459=CARTESIAN_POINT ( 'NONE',  ( 0.000000000000000000, 20.00000000000000000, 0.000000000000000000 ) ) ;
#8466=CARTESIAN_POINT ( 'NONE',  ( -4.458734124999999437, -26.18750000136559919, -5.460374474430324690E-16 ) ) ;
#8470=VERTEX_POINT ( 'NONE', #12668 ) ;
#8471=ORIENTED_EDGE ( 'NONE', *, *, #5019, .F. ) ;
#8473=CARTESIAN_POINT ( 'NONE',  ( -1.846868145590734756, -24.37500000136559564, -4.458734125000000326 ) ) ;
#8480=CARTESIAN_POINT ( 'NONE',  ( -3.535533905932737309, -22.62500000000000000, -3.535533905932738197 ) ) ;
#8487=CARTESIAN_POINT ( 'NONE',  ( 4.458734124999999437, -28.43750000136559564, 0.000000000000000000 ) ) ;
#8494=DIRECTION ( 'NONE',  ( 1.239088197126290570E-16, -0.000000000000000000, 1.000000000000000000 ) ) ;
#8496=CARTESIAN_POINT ( 'NONE',  ( 1.846868145590736310, -23.62500000136559919, 4.458734124999999437 ) ) ;
#8498=ORIENTED_EDGE ( 'NONE', *, *, #1935, .F. ) ;
#8503=CARTESIAN_POINT ( 'NONE',  ( 3.535533905932736864, -22.12500000000000000, 3.535533905932738641 ) ) ;
#8506=CARTESIAN_POINT ( 'NONE',  ( 3.152801135295366208, -21.81250000136559208, 3.152801135295367985 ) ) ;
#8517=ORIENTED_EDGE ( 'NONE', *, *, #3556, .T. ) ;
#8538=CARTESIAN_POINT ( 'NONE',  ( -9.184850993605147944E-16, -27.37500000273118772, 5.000000000000000000 ) ) ;
#8539=DIRECTION ( 'NONE',  ( 0.000000000000000000, 1.000000000000000000, 0.000000000000000000 ) ) ;
#8541=EDGE_CURVE ( 'NONE', #2810, #8470, #7955, .T. ) ;
#8543=CARTESIAN_POINT ( 'NONE',  ( 0.000000000000000000, -20.00000000000000000, 0.000000000000000000 ) ) ;
#8546=CARTESIAN_POINT ( 'NONE',  ( 1.846868145590736310, -25.87500000136559564, 4.458734124999997661 ) ) ;
#8547=CARTESIAN_POINT ( 'NONE',  ( 4.458734124999999437, -22.37500000136559564, -1.846868145590734978 ) ) ;
#8551=ORIENTED_EDGE ( 'NONE', *, *, #7275, .T. ) ;
#8553=CARTESIAN_POINT ( 'NONE',  ( 1.846868145590736310, -22.87500000136559564, 4.458734124999999437 ) ) ;
#8554=CYLINDRICAL_SURFACE ( 'NONE', #7915, 2.649999999999992806 ) ;
#8558=DIRECTION ( 'NONE',  ( 0.000000000000000000, 1.000000000000000000, 0.000000000000000000 ) ) ;
#8559=CARTESIAN_POINT ( 'NONE',  ( 3.535533905932738197, -22.87500000000000000, -3.535533905932738197 ) ) ;
#8563=CARTESIAN_POINT ( 'NONE',  ( -4.458734125000000326, -26.00000000136559208, -1.846868145590735644 ) ) ;
#8570=CARTESIAN_POINT ( 'NONE',  ( -4.458734125000000326, -24.00000000136559564, -1.846868145590735644 ) ) ;
#8573=DIRECTION ( 'NONE',  ( -0.000000000000000000, 1.000000000000000000, -0.000000000000000000 ) ) ;
#8579=CARTESIAN_POINT ( 'NONE',  ( 4.458734124999999437, -21.68750000136559208, 0.000000000000000000 ) ) ;
#8583=CARTESIAN_POINT ( 'NONE',  ( -2.071067811865475061, -27.81250000273118772, -5.000000000000000888 ) ) ;
#8585=CARTESIAN_POINT ( 'NONE',  ( -3.152801135295367985, -30.81250000136559564, 3.152801135295367096 ) ) ;
#8589=DIRECTION ( 'NONE',  ( 0.000000000000000000, 1.000000000000000000, 0.000000000000000000 ) ) ;
#8592=EDGE_CURVE ( 'NONE', #9570, #2381, #5803, .T. ) ;
#8616=CARTESIAN_POINT ( 'NONE',  ( -5.000000000000000888, -30.68750000273118772, -2.071067811865475949 ) ) ;
#8619=CARTESIAN_POINT ( 'NONE',  ( -4.458734124999999437, -24.18750000136559564, -5.460374474430324690E-16 ) ) ;
#8620=CARTESIAN_POINT ( 'NONE',  ( 3.152801135295367541, -22.31250000136559564, -3.152801135295367541 ) ) ;
#8625=( BOUNDED_CURVE ( )  B_SPLINE_CURVE ( 2, ( #7142, #12045, #5924, #4543, #15713, #14413, #2275, #10922, #4628 ),
 .UNSPECIFIED., .F., .F. ) 
 B_SPLINE_CURVE_WITH_KNOTS ( ( 3, 2, 2, 2, 3 ),
 ( 0.5250000000000001332, 0.5375000000000000888, 0.5500000000000000444, 0.5625000000000000000, 0.5749999999999998446 ),
 .UNSPECIFIED. ) 
 CURVE ( )  GEOMETRIC_REPRESENTATION_ITEM ( )  RATIONAL_B_SPLINE_CURVE ( ( 0.9999999999999993339, 0.9238795325112874046, 1.000000000000000000, 0.9238795325112867385, 1.000000000000000000, 0.9238795325112867385, 1.000000000000000000, 0.9238795325112874046, 0.9999999999999993339 ) ) 
 REPRESENTATION_ITEM ( '' )  );
#8627=ORIENTED_EDGE ( 'NONE', *, *, #8541, .T. ) ;
#8628=CARTESIAN_POINT ( 'NONE',  ( 4.458734124999999437, -21.68750000136559208, 0.000000000000000000 ) ) ;
#8631=CARTESIAN_POINT ( 'NONE',  ( -2.071067811865468400, -27.81250000273118772, -5.000000000000007994 ) ) ;
#8635=CARTESIAN_POINT ( 'NONE',  ( -5.000000000000000888, -23.43749999999999645, 2.071067811865474617 ) ) ;
#8638=CARTESIAN_POINT ( 'NONE',  ( 4.458734124999999437, -28.50000000136559564, 1.846868145590737864 ) ) ;
#8646=CARTESIAN_POINT ( 'NONE',  ( -4.458734125000000326, -23.00000000136559564, -1.846868145590735644 ) ) ;
#8649=EDGE_LOOP ( 'NONE', ( #15044, #4484, #270, #14984 ) ) ;
#8655=CARTESIAN_POINT ( 'NONE',  ( -4.458734125000000326, -25.25000000136559564, -1.846868145590735644 ) ) ;
#8658=CARTESIAN_POINT ( 'NONE',  ( -3.535533905932737309, -27.75000000273118772, -3.535533905932738197 ) ) ;
#8661=CARTESIAN_POINT ( 'NONE',  ( 2.730187237215162345E-16, -30.18750000136559564, -4.458734124999999437 ) ) ;
#8664=ORIENTED_EDGE ( 'NONE', *, *, #3327, .T. ) ;
#8666=CIRCLE ( 'NONE', #1689, 25.00000000000000000 ) ;
#8668=DIRECTION ( 'NONE',  ( -0.8660254037844410391, 0.4999999999999958367, -0.000000000000000000 ) ) ;
#8669=AXIS2_PLACEMENT_3D ( 'NONE', #5921, #10844, #14556 ) ;
#8684=EDGE_LOOP ( 'NONE', ( #14969, #4952, #3010, #583 ) ) ;
#8690=DIRECTION ( 'NONE',  ( -0.000000000000000000, 1.000000000000000000, -0.000000000000000000 ) ) ;
#8692=CARTESIAN_POINT ( 'NONE',  ( 2.071067811865476394, -27.31250000273118772, 5.000000000000000000 ) ) ;
#8694=CARTESIAN_POINT ( 'NONE',  ( -3.535533905932737309, -24.62500000000000000, -3.535533905932738197 ) ) ;
#8696=AXIS2_PLACEMENT_3D ( 'NONE', #12162, #1100, #2462 ) ;
#8698=CARTESIAN_POINT ( 'NONE',  ( -1.846868145590737420, -25.00000000136559564, 4.458734124999997661 ) ) ;
#8701=CARTESIAN_POINT ( 'NONE',  ( -4.458734124999999437, -24.00000000136559564, -1.846868145590735644 ) ) ;
#8709=CARTESIAN_POINT ( 'NONE',  ( 4.458734124999999437, -21.75000000136559564, 1.846868145590737864 ) ) ;
#8720=CARTESIAN_POINT ( 'NONE',  ( -3.152801135295367096, -26.06250000136559564, -3.152801135295367541 ) ) ;
#8727=EDGE_LOOP ( 'NONE', ( #6944, #2012 ) ) ;
#8728=VERTEX_POINT ( 'NONE', #3530 ) ;
#8730=CARTESIAN_POINT ( 'NONE',  ( -8.190561711645485556E-16, -26.68750000136559564, 4.458734124999999437 ) ) ;
#8735=DIRECTION ( 'NONE',  ( -0.000000000000000000, 1.000000000000000000, -0.000000000000000000 ) ) ;
#8739=CARTESIAN_POINT ( 'NONE',  ( -5.000000000000000888, -29.56250000000000355, -2.071067811865475949 ) ) ;
#8742=CARTESIAN_POINT ( 'NONE',  ( -3.535533905932737309, -26.75000000273118772, -3.535533905932738197 ) ) ;
#8743=EDGE_CURVE ( 'NONE', #3154, #14037, #3561, .T. ) ;
#8746=CARTESIAN_POINT ( 'NONE',  ( 5.000000000000000000, -24.18750000273119127, 2.071067811865478614 ) ) ;
#8750=ORIENTED_EDGE ( 'NONE', *, *, #6097, .T. ) ;
#8755=DIRECTION ( 'NONE',  ( -0.000000000000000000, -1.000000000000000000, -0.000000000000000000 ) ) ;
#8760=AXIS2_PLACEMENT_3D ( 'NONE', #10106, #13967, #5336 ) ;
#8764=DIRECTION ( 'NONE',  ( 0.000000000000000000, 0.000000000000000000, 1.000000000000000000 ) ) ;
#8769=CARTESIAN_POINT ( 'NONE',  ( 3.152801135295367541, -31.31250000136559564, -3.152801135295367541 ) ) ;
#8772=CARTESIAN_POINT ( 'NONE',  ( -9.184850993605147944E-16, -27.25000000000000000, 5.000000000000000000 ) ) ;
#8774=EDGE_CURVE ( 'NONE', #10093, #6661, #1105, .T. ) ;
#8778=CARTESIAN_POINT ( 'NONE',  ( -3.535533905932738641, -30.50000000273118772, 3.535533905932737309 ) ) ;
#8780=CARTESIAN_POINT ( 'NONE',  ( 35.00000000000000000, 40.00000000000000000, -8.572527594031472993E-15 ) ) ;
#8782=CARTESIAN_POINT ( 'NONE',  ( 3.152801135295366208, -25.81250000136559564, 3.152801135295367985 ) ) ;
#8790=CARTESIAN_POINT ( 'NONE',  ( -1.846868145590734756, -22.37500000136559564, -4.458734125000000326 ) ) ;
#8792=CARTESIAN_POINT ( 'NONE',  ( -2.071067811865478170, -27.43750000273119127, 5.000000000000000000 ) ) ;
#8800=CARTESIAN_POINT ( 'NONE',  ( -3.152801135295367985, -25.81250000136559564, 3.152801135295367096 ) ) ;
#8807=CARTESIAN_POINT ( 'NONE',  ( 4.458734124999999437, -24.43750000136559564, 0.000000000000000000 ) ) ;
#8811=EDGE_CURVE ( 'NONE', #15000, #14496, #11202, .T. ) ;
#8818=( BOUNDED_CURVE ( )  B_SPLINE_CURVE ( 2, ( #15201, #1691, #14458, #10740, #961, #2086, #15760, #5886, #15445 ),
 .UNSPECIFIED., .F., .F. ) 
 B_SPLINE_CURVE_WITH_KNOTS ( ( 3, 2, 2, 2, 3 ),
 ( 0.9249999999999998224, 0.9374999999999997780, 0.9499999999999998446, 0.9624999999999999112, 0.9749999999999998668 ),
 .UNSPECIFIED. ) 
 CURVE ( )  GEOMETRIC_REPRESENTATION_ITEM ( )  RATIONAL_B_SPLINE_CURVE ( ( 1.000000000000001332, 0.9238795325112854062, 1.000000000000000000, 0.9238795325112867385, 1.000000000000000000, 0.9238795325112867385, 1.000000000000000000, 0.9238795325112874046, 0.9999999999999993339 ) ) 
 REPRESENTATION_ITEM ( '' )  );
#8819=CARTESIAN_POINT ( 'NONE',  ( 5.000000000000000888, -31.93750000000000355, -2.071067811865475505 ) ) ;
#8822=CARTESIAN_POINT ( 'NONE',  ( 5.000000000000000888, -29.06250000273118772, -2.071067811865475505 ) ) ;
#8824=CARTESIAN_POINT ( 'NONE',  ( -4.458734124999999437, -28.93750000136559564, -5.460374474430324690E-16 ) ) ;
#8832=EDGE_CURVE ( 'NONE', #9262, #10619, #4987, .T. ) ;
#8833=CARTESIAN_POINT ( 'NONE',  ( 0.000000000000000000, 20.00000000000000000, 25.00000000000000000 ) ) ;
#8842=ORIENTED_EDGE ( 'NONE', *, *, #7794, .F. ) ;
#8856=DIRECTION ( 'NONE',  ( 0.000000000000000000, 0.000000000000000000, -1.000000000000000000 ) ) ;
#8857=LINE ( 'NONE', #15156, #13022 ) ;
#8866=ORIENTED_EDGE ( 'NONE', *, *, #6987, .F. ) ;
#8867=CARTESIAN_POINT ( 'NONE',  ( 4.769696007084728073, -13.00000000000000178, -1.500000000000000000 ) ) ;
#8869=CARTESIAN_POINT ( 'NONE',  ( 24.26932219902320043, 20.00000000000000000, 5.999999999999992895 ) ) ;
#8872=CARTESIAN_POINT ( 'NONE',  ( -35.00000000000000000, 37.00000000000000000, 0.000000000000000000 ) ) ;
#8875=CARTESIAN_POINT ( 'NONE',  ( 3.535533905932738197, -29.87500000000000000, -3.535533905932738197 ) ) ;
#8877=CARTESIAN_POINT ( 'NONE',  ( 3.152801135295366208, -24.56250000136559564, 3.152801135295367985 ) ) ;
#8887=CARTESIAN_POINT ( 'NONE',  ( 3.152801135295367541, -22.31250000136559564, -3.152801135295367541 ) ) ;
#8888=LINE ( 'NONE', #13790, #1704 ) ;
#8895=CARTESIAN_POINT ( 'NONE',  ( -3.535533905932738641, -29.37500000000000355, 3.535533905932737309 ) ) ;
#8898=CARTESIAN_POINT ( 'NONE',  ( 3.061616997868383141E-16, -27.87500000273118772, -5.000000000000000000 ) ) ;
#8901=CARTESIAN_POINT ( 'NONE',  ( -3.152801135295367985, -29.81250000136559208, 3.152801135295367096 ) ) ;
#8915=CARTESIAN_POINT ( 'NONE',  ( -2.071067811865477726, -31.68750000000000000, -4.999999999999996447 ) ) ;
#8918=CARTESIAN_POINT ( 'NONE',  ( 5.000000000000000000, -22.00000000000000000, 0.000000000000000000 ) ) ;
#8920=LINE ( 'NONE', #7631, #6107 ) ;
#8928=AXIS2_PLACEMENT_3D ( 'NONE', #3339, #9557, #9708 ) ;
#8935=CARTESIAN_POINT ( 'NONE',  ( 2.071067811865468844, -26.93750000273118772, -5.000000000000007994 ) ) ;
#8940=CARTESIAN_POINT ( 'NONE',  ( 35.00000000000000000, 37.00000000000000000, -8.572527594031472993E-15 ) ) ;
#8951=DIRECTION ( 'NONE',  ( 0.000000000000000000, 1.000000000000000000, 0.000000000000000000 ) ) ;
#8959=DIRECTION ( 'NONE',  ( -0.000000000000000000, 1.000000000000000000, -0.000000000000000000 ) ) ;
#8961=CARTESIAN_POINT ( 'NONE',  ( 1.846868145590736310, -22.62500000136559564, 4.458734124999999437 ) ) ;
#8964=ORIENTED_EDGE ( 'NONE', *, *, #5448, .T. ) ;
#8967=VERTEX_POINT ( 'NONE', #15422 ) ;
#8968=CARTESIAN_POINT ( 'NONE',  ( 2.730187237215162345E-16, -31.43750000136559564, -4.458734124999999437 ) ) ;
#8975=EDGE_CURVE ( 'NONE', #4620, #12657, #4695, .T. ) ;
#8979=CARTESIAN_POINT ( 'NONE',  ( 2.071067811865475505, -29.81249999999999645, -5.000000000000000888 ) ) ;
#8983=CARTESIAN_POINT ( 'NONE',  ( -2.071067811865475061, -22.81250000273118417, -5.000000000000000888 ) ) ;
#8985=CARTESIAN_POINT ( 'NONE',  ( 3.152801135295367541, -28.31250000136559564, -3.152801135295367541 ) ) ;
#8999=CARTESIAN_POINT ( 'NONE',  ( 4.458734124999999437, -30.75000000136559564, 1.846868145590737864 ) ) ;
#9025=DIRECTION ( 'NONE',  ( 0.000000000000000000, 1.000000000000000000, 0.000000000000000000 ) ) ;
#9034=ORIENTED_EDGE ( 'NONE', *, *, #6721, .T. ) ;
#9046=CARTESIAN_POINT ( 'NONE',  ( -1.846868145590737420, -24.75000000136559564, 4.458734124999999437 ) ) ;
#9052=EDGE_LOOP ( 'NONE', ( #7783, #12254, #6339 ) ) ;
#9053=CARTESIAN_POINT ( 'NONE',  ( 4.458734124999999437, -29.68750000136559208, 0.000000000000000000 ) ) ;
#9062=CARTESIAN_POINT ( 'NONE',  ( -5.000000000000000888, -31.56249999999999645, -2.071067811865475949 ) ) ;
#9066=CARTESIAN_POINT ( 'NONE',  ( -5.000000000000000888, -24.68750000273118772, -2.071067811865475949 ) ) ;
#9068=CARTESIAN_POINT ( 'NONE',  ( -4.458734124999999437, -28.00000000136559564, -1.846868145590735644 ) ) ;
#9076=VERTEX_POINT ( 'NONE', #9353 ) ;
#9077=DIRECTION ( 'NONE',  ( -0.000000000000000000, -1.000000000000000000, -0.000000000000000000 ) ) ;
#9078=CARTESIAN_POINT ( 'NONE',  ( 0.000000000000000000, -20.00000000000000000, 0.000000000000000000 ) ) ;
#9093=CARTESIAN_POINT ( 'NONE',  ( 35.00000000000000000, 37.00000000000000000, -8.572527594031472993E-15 ) ) ;
#9096=CARTESIAN_POINT ( 'NONE',  ( -3.535533905932738641, -23.37500000000000000, 3.535533905932737309 ) ) ;
#9097=FACE_OUTER_BOUND ( 'NONE', #7161, .T. ) ;
#9098=CARTESIAN_POINT ( 'NONE',  ( 2.730187237215162345E-16, -22.43750000136559564, -4.458734124999999437 ) ) ;
#9100=DIRECTION ( 'NONE',  ( 0.000000000000000000, 1.000000000000000000, 0.000000000000000000 ) ) ;
#9103=EDGE_CURVE ( 'NONE', #13770, #14954, #8028, .T. ) ;
#9108=EDGE_CURVE ( 'NONE', #3157, #3489, #3816, .T. ) ;
#9121=CARTESIAN_POINT ( 'NONE',  ( 4.458734125000000326, -24.37500000136559564, -1.846868145590734978 ) ) ;
#9123=ORIENTED_EDGE ( 'NONE', *, *, #11925, .F. ) ;
#9129=CARTESIAN_POINT ( 'NONE',  ( -4.458734125000000326, -31.25000000136559564, -1.846868145590735644 ) ) ;
#9137=CARTESIAN_POINT ( 'NONE',  ( -5.000000000000000888, -27.56250000000000000, -2.071067811865475949 ) ) ;
#9142=CARTESIAN_POINT ( 'NONE',  ( 5.000000000000000000, -25.18750000273119127, 2.071067811865478614 ) ) ;
#9144=CARTESIAN_POINT ( 'NONE',  ( 4.458734124999999437, -25.37500000136559564, -1.846868145590734978 ) ) ;
#9154=CYLINDRICAL_SURFACE ( 'NONE', #10402, 5.000000000000000000 ) ;
#9155=CARTESIAN_POINT ( 'NONE',  ( 4.458734124999999437, -27.75000000136559564, 1.846868145590737864 ) ) ;
#9163=ORIENTED_EDGE ( 'NONE', *, *, #6286, .F. ) ;
#9164=CARTESIAN_POINT ( 'NONE',  ( 1.846868145590736310, -29.62500000136559208, 4.458734124999999437 ) ) ;
#9168=DIRECTION ( 'NONE',  ( 0.000000000000000000, 1.000000000000000000, 0.000000000000000000 ) ) ;
#9169=EDGE_CURVE ( 'NONE', #7938, #8470, #13600, .T. ) ;
#9177=CARTESIAN_POINT ( 'NONE',  ( 4.458734124999997661, -23.75000000136559564, 1.846868145590737864 ) ) ;
#9179=CIRCLE ( 'NONE', #6078, 6.000000000000000888 ) ;
#9180=LINE ( 'NONE', #1968, #15174 ) ;
#9182=CARTESIAN_POINT ( 'NONE',  ( -9.184850993605147944E-16, -26.37500000273118417, 5.000000000000000000 ) ) ;
#9195=DIRECTION ( 'NONE',  ( 0.000000000000000000, 0.000000000000000000, -1.000000000000000000 ) ) ;
#9198=CARTESIAN_POINT ( 'NONE',  ( 35.00000000000000000, 40.00000000000000000, 5.999999999999991118 ) ) ;
#9201=CARTESIAN_POINT ( 'NONE',  ( 4.458734124999999437, -21.43750000136559208, 0.000000000000000000 ) ) ;
#9203=VERTEX_POINT ( 'NONE', #2614 ) ;
#9208=CARTESIAN_POINT ( 'NONE',  ( 4.458734124999999437, -29.75000000136559564, 1.846868145590737864 ) ) ;
#9211=CARTESIAN_POINT ( 'NONE',  ( -9.184850993605147944E-16, -28.25000000000000000, 5.000000000000000000 ) ) ;
#9216=EDGE_CURVE ( 'NONE', #2292, #10237, #4081, .T. ) ;
#9217=CARTESIAN_POINT ( 'NONE',  ( 5.000000000000000000, -25.00000000000000000, 0.000000000000000000 ) ) ;
#9219=PLANE ( 'NONE',  #13501 ) ;
#9221=CARTESIAN_POINT ( 'NONE',  ( 5.000000000000000888, -25.06250000273118417, -2.071067811865475505 ) ) ;
#9223=CARTESIAN_POINT ( 'NONE',  ( -1.846868145590737420, -25.75000000136559564, 4.458734124999997661 ) ) ;
#9231=VECTOR ( 'NONE', #4207, 1000.000000000000000 ) ;
#9237=CARTESIAN_POINT ( 'NONE',  ( 4.458734124999999437, -28.68750000136559564, 0.000000000000000000 ) ) ;
#9262=VERTEX_POINT ( 'NONE', #2532 ) ;
#9265=ORIENTED_EDGE ( 'NONE', *, *, #10379, .F. ) ;
#9272=ADVANCED_FACE ( 'NONE', ( #9097 ), #6677, .F. ) ;
#9275=VECTOR ( 'NONE', #7481, 1000.000000000000000 ) ;
#9277=CARTESIAN_POINT ( 'NONE',  ( 3.061616997868383141E-16, -25.75000000000000355, -5.000000000000000000 ) ) ;
#9280=CARTESIAN_POINT ( 'NONE',  ( 35.00000000000000000, 40.00000000000000000, -5.999999999999991118 ) ) ;
#9281=VECTOR ( 'NONE', #5595, 1000.000000000000114 ) ;
#9283=CARTESIAN_POINT ( 'NONE',  ( 4.458734124999999437, -31.62500000136559564, -1.846868145590734978 ) ) ;
#9286=ORIENTED_EDGE ( 'NONE', *, *, #11418, .T. ) ;
#9288=ORIENTED_EDGE ( 'NONE', *, *, #14488, .T. ) ;
#9290=CARTESIAN_POINT ( 'NONE',  ( -3.152801135295367096, -25.31250000136559564, -3.152801135295367541 ) ) ;
#9299=CARTESIAN_POINT ( 'NONE',  ( 3.535533905932738197, -25.87500000000000355, -3.535533905932738197 ) ) ;
#9303=CARTESIAN_POINT ( 'NONE',  ( -5.000000000000000888, -23.56250000273118417, 2.071067811865474617 ) ) ;
#9305=CARTESIAN_POINT ( 'NONE',  ( 1.846868145590735200, -26.25000000136559564, -4.458734124999999437 ) ) ;
#9307=ORIENTED_EDGE ( 'NONE', *, *, #2866, .T. ) ;
#9317=CARTESIAN_POINT ( 'NONE',  ( 4.458734124999999437, -27.68750000136559564, 0.000000000000000000 ) ) ;
#9324=CARTESIAN_POINT ( 'NONE',  ( 0.000000000000000000, -20.00000000000000000, 0.000000000000000000 ) ) ;
#9327=CARTESIAN_POINT ( 'NONE',  ( 5.000000000000000000, -21.56250000136559208, 0.000000000000000000 ) ) ;
#9333=SURFACE_STYLE_USAGE ( .BOTH. , #6585 ) ;
#9336=DIRECTION ( 'NONE',  ( 0.000000000000000000, -1.000000000000000000, 0.000000000000000000 ) ) ;
#9345=DIRECTION ( 'NONE',  ( 0.000000000000000000, 1.000000000000000000, 0.000000000000000000 ) ) ;
#9346=MANIFOLD_SOLID_BREP ( 'M5 Clearance Hole1', #13312 ) ;
#9347=CARTESIAN_POINT ( 'NONE',  ( 2.071067811865461294, -25.93750000273118062, -5.000000000000014211 ) ) ;
#9353=CARTESIAN_POINT ( 'NONE',  ( 3.061616997868383141E-16, -23.87500000273118772, -5.000000000000000000 ) ) ;
#9355=CARTESIAN_POINT ( 'NONE',  ( 3.152801135295366208, -28.81250000136559564, 3.152801135295367985 ) ) ;
#9362=CARTESIAN_POINT ( 'NONE',  ( 4.458734124999999437, -28.68750000136559564, 0.000000000000000000 ) ) ;
#9370=CARTESIAN_POINT ( 'NONE',  ( -9.184850993605147944E-16, -24.25000000000000000, 5.000000000000000000 ) ) ;
#9372=CARTESIAN_POINT ( 'NONE',  ( 6.123233995736766282E-16, 20.00000000000000000, -5.000000000000000000 ) ) ;
#9376=CARTESIAN_POINT ( 'NONE',  ( 4.458734125000000326, -30.37500000136559564, -1.846868145590734978 ) ) ;
#9385=ORIENTED_EDGE ( 'NONE', *, *, #1140, .T. ) ;
#9388=CARTESIAN_POINT ( 'NONE',  ( 4.458734125000000326, -27.62500000136559564, -1.846868145590734978 ) ) ;
#9405=EDGE_CURVE ( 'NONE', #14954, #11629, #5740, .T. ) ;
#9411=FACE_OUTER_BOUND ( 'NONE', #10687, .T. ) ;
#9416=LINE ( 'NONE', #929, #1760 ) ;
#9418=AXIS2_PLACEMENT_3D ( 'NONE', #11670, #9345, #7984 ) ;
#9420=CARTESIAN_POINT ( 'NONE',  ( 5.000000000000000000, -23.18750000273119127, 2.071067811865478614 ) ) ;
#9425=VECTOR ( 'NONE', #680, 1000.000000000000000 ) ;
#9431=CARTESIAN_POINT ( 'NONE',  ( -1.846868145590734756, -30.37500000136559564, -4.458734124999999437 ) ) ;
#9435=VERTEX_POINT ( 'NONE', #6993 ) ;
#9439=CARTESIAN_POINT ( 'NONE',  ( -4.458734124999999437, -27.18750000136559564, -5.460374474430324690E-16 ) ) ;
#9443=CARTESIAN_POINT ( 'NONE',  ( -3.535533905932738641, -29.37500000000000355, 3.535533905932737309 ) ) ;
#9446=CARTESIAN_POINT ( 'NONE',  ( 5.000000000000000000, -27.00000000000000000, 0.000000000000000000 ) ) ;
#9450=CARTESIAN_POINT ( 'NONE',  ( -4.458734125000001214, -29.87500000136559564, 1.846868145590734089 ) ) ;
#9451=AXIS2_PLACEMENT_3D ( 'NONE', #13210, #4741, #12321 ) ;
#9453=CARTESIAN_POINT ( 'NONE',  ( -4.458734124999999437, -23.00000000136559564, -1.846868145590735644 ) ) ;
#9458=CARTESIAN_POINT ( 'NONE',  ( -4.458734124999999437, -26.93750000136559564, -5.460374474430324690E-16 ) ) ;
#9464=AXIS2_PLACEMENT_3D ( 'NONE', #14759, #1097, #7332 ) ;
#9466=CARTESIAN_POINT ( 'NONE',  ( -1.846868145590737420, -28.00000000136559564, 4.458734124999999437 ) ) ;
#9492=CARTESIAN_POINT ( 'NONE',  ( 0.000000000000000000, -32.00000000000000000, 0.000000000000000000 ) ) ;
#9509=CARTESIAN_POINT ( 'NONE',  ( 1.846868145590736310, -30.87500000136559564, 4.458734124999997661 ) ) ;
#9519=CARTESIAN_POINT ( 'NONE',  ( 4.458734124999999437, -26.75000000136559564, 1.846868145590737864 ) ) ;
#9520=CARTESIAN_POINT ( 'NONE',  ( 3.061616997868383141E-16, -23.87500000273118772, -5.000000000000000000 ) ) ;
#9527=CARTESIAN_POINT ( 'NONE',  ( -5.000000000000000888, -23.56250000000000000, -2.071067811865475949 ) ) ;
#9531=CARTESIAN_POINT ( 'NONE',  ( 5.000000000000000000, -22.12500000273118417, 0.000000000000000000 ) ) ;
#9534=ADVANCED_FACE ( 'NONE', ( #10050 ), #14809, .T. ) ;
#9539=CARTESIAN_POINT ( 'NONE',  ( -3.152801135295367985, -27.81250000136559564, 3.152801135295367096 ) ) ;
#9545=DIRECTION ( 'NONE',  ( 0.000000000000000000, 1.000000000000000000, 0.000000000000000000 ) ) ;
#9546=CARTESIAN_POINT ( 'NONE',  ( 3.152801135295366208, -23.81250000136559564, 3.152801135295367985 ) ) ;
#9547=CARTESIAN_POINT ( 'NONE',  ( 0.000000000000000000, 20.00000000000000000, 0.000000000000000000 ) ) ;
#9557=DIRECTION ( 'NONE',  ( 0.000000000000000000, 1.000000000000000000, 0.000000000000000000 ) ) ;
#9562=LINE ( 'NONE', #8365, #12313 ) ;
#9566=CARTESIAN_POINT ( 'NONE',  ( -2.071067811865503483, -22.68750000000000000, -4.999999999999971578 ) ) ;
#9568=CARTESIAN_POINT ( 'NONE',  ( 5.000000000000000000, -32.00000000000000000, 0.000000000000000000 ) ) ;
#9570=VERTEX_POINT ( 'NONE', #13489 ) ;
#9572=DIRECTION ( 'NONE',  ( 0.000000000000000000, 1.000000000000000000, 0.000000000000000000 ) ) ;
#9575=CARTESIAN_POINT ( 'NONE',  ( 6.000000000000000000, -20.00000000000000000, 1.500000000000000000 ) ) ;
#9578=EDGE_CURVE ( 'NONE', #2190, #1108, #15657, .T. ) ;
#9580=CARTESIAN_POINT ( 'NONE',  ( -4.458734124999999437, -31.25000000136559564, -1.846868145590735644 ) ) ;
#9584=CARTESIAN_POINT ( 'NONE',  ( 35.00000000000000000, 37.00000000000000000, -8.572527594031472993E-15 ) ) ;
#9588=CARTESIAN_POINT ( 'NONE',  ( 3.152801135295367541, -28.56250000136559564, -3.152801135295367541 ) ) ;
#9590=CARTESIAN_POINT ( 'NONE',  ( 3.061616997868383141E-16, -29.87500000273118417, -5.000000000000000000 ) ) ;
#9593=CARTESIAN_POINT ( 'NONE',  ( 3.535533905932738197, -23.87500000000000000, -3.535533905932738197 ) ) ;
#9597=CARTESIAN_POINT ( 'NONE',  ( -4.458734125000000326, -31.00000000136559564, -1.846868145590735644 ) ) ;
#9604=CARTESIAN_POINT ( 'NONE',  ( 4.458734124999999437, -27.43750000136559564, 0.000000000000000000 ) ) ;
#9612=CARTESIAN_POINT ( 'NONE',  ( -8.190561711645485556E-16, -24.93750000136559564, 4.458734124999999437 ) ) ;
#9616=CIRCLE ( 'NONE', #2124, 25.00000000000000000 ) ;
#9621=ORIENTED_EDGE ( 'NONE', *, *, #4689, .T. ) ;
#9626=EDGE_CURVE ( 'NONE', #13586, #2123, #10181, .T. ) ;
#9634=VERTEX_POINT ( 'NONE', #15773 ) ;
#9635=CARTESIAN_POINT ( 'NONE',  ( -3.535533905932738641, -22.37500000000000000, 3.535533905932737309 ) ) ;
#9651=CARTESIAN_POINT ( 'NONE',  ( 2.730187237215162345E-16, -24.43750000136559564, -4.458734124999999437 ) ) ;
#9660=DIRECTION ( 'NONE',  ( 0.000000000000000000, 0.000000000000000000, -1.000000000000000000 ) ) ;
#9662=CARTESIAN_POINT ( 'NONE',  ( 2.071067811865485275, -30.31250000273118062, 4.999999999999989342 ) ) ;
#9665=AXIS2_PLACEMENT_3D ( 'NONE', #15254, #311, #11284 ) ;
#9672=CARTESIAN_POINT ( 'NONE',  ( 3.152801135295367541, -30.31250000136559564, -3.152801135295367541 ) ) ;
#9680=FACE_OUTER_BOUND ( 'NONE', #1460, .T. ) ;
#9681=CARTESIAN_POINT ( 'NONE',  ( -1.846868145590734756, -30.12500000136559208, -4.458734125000000326 ) ) ;
#9682=CARTESIAN_POINT ( 'NONE',  ( 0.000000000000000000, -13.00000000000000178, 0.000000000000000000 ) ) ;
#9683=ORIENTED_EDGE ( 'NONE', *, *, #2620, .F. ) ;
#9685=ADVANCED_FACE ( 'NONE', ( #899 ), #13465, .T. ) ;
#9692=CARTESIAN_POINT ( 'NONE',  ( -1.846868145590737420, -22.00000000136559208, 4.458734124999999437 ) ) ;
#9708=DIRECTION ( 'NONE',  ( 0.000000000000000000, 0.000000000000000000, 1.000000000000000000 ) ) ;
#9710=CARTESIAN_POINT ( 'NONE',  ( -5.000000000000000888, -25.56250000273118417, 2.071067811865474617 ) ) ;
#9718=CARTESIAN_POINT ( 'NONE',  ( -9.184850993605147944E-16, -21.37500000273118772, 5.000000000000000000 ) ) ;
#9719=( NAMED_UNIT ( * ) PLANE_ANGLE_UNIT ( ) SI_UNIT ( $, .RADIAN. ) );
#9724=ORIENTED_EDGE ( 'NONE', *, *, #10590, .T. ) ;
#9727=EDGE_CURVE ( 'NONE', #10564, #3510, #11226, .T. ) ;
#9731=AXIS2_PLACEMENT_3D ( 'NONE', #13926, #8690, #3906 ) ;
#9735=CARTESIAN_POINT ( 'NONE',  ( -5.000000000000000888, -22.56250000273118772, 2.071067811865474617 ) ) ;
#9736=CARTESIAN_POINT ( 'NONE',  ( -4.458734124999999437, -25.25000000136559564, -1.846868145590735644 ) ) ;
#9740=EDGE_CURVE ( 'NONE', #2783, #2143, #10039, .T. ) ;
#9746=ORIENTED_EDGE ( 'NONE', *, *, #13573, .F. ) ;
#9747=CARTESIAN_POINT ( 'NONE',  ( -4.458734125000001214, -22.12500000136559564, 1.846868145590734089 ) ) ;
#9759=CARTESIAN_POINT ( 'NONE',  ( 1.846868145590736310, -27.62500000136559564, 4.458734124999999437 ) ) ;
#9767=CARTESIAN_POINT ( 'NONE',  ( 0.000000000000000000, -20.00000000000000000, 0.000000000000000000 ) ) ;
#9769=CARTESIAN_POINT ( 'NONE',  ( 4.458734125000000326, -23.37500000136559564, -1.846868145590734978 ) ) ;
#9772=FACE_OUTER_BOUND ( 'NONE', #2325, .T. ) ;
#9780=CARTESIAN_POINT ( 'NONE',  ( 4.458734124999999437, -21.75000000136559564, 1.846868145590737864 ) ) ;
#9783=CARTESIAN_POINT ( 'NONE',  ( -2.071067811865475061, -29.81250000273118417, -5.000000000000000888 ) ) ;
#9786=EDGE_CURVE ( 'NONE', #9076, #1108, #1603, .T. ) ;
#9787=CARTESIAN_POINT ( 'NONE',  ( 3.535533905932738197, -24.87500000000000000, -3.535533905932738197 ) ) ;
#9796=ORIENTED_EDGE ( 'NONE', *, *, #13213, .T. ) ;
#9799=CARTESIAN_POINT ( 'NONE',  ( -2.071067811865450192, -25.43750000273118062, 5.000000000000028422 ) ) ;
#9818=CARTESIAN_POINT ( 'NONE',  ( -5.000000000000000888, -24.43750000000000355, 2.071067811865474617 ) ) ;
#9820=CARTESIAN_POINT ( 'NONE',  ( 3.152801135295367541, -25.56250000136559564, -3.152801135295367541 ) ) ;
#9821=CARTESIAN_POINT ( 'NONE',  ( -8.190561711645485556E-16, -23.68750000136559564, 4.458734124999999437 ) ) ;
#9828=CARTESIAN_POINT ( 'NONE',  ( 3.152801135295367541, -23.56250000136559564, -3.152801135295367541 ) ) ;
#9831=PLANE ( 'NONE',  #8696 ) ;
#9834=CARTESIAN_POINT ( 'NONE',  ( 5.000000000000000000, -22.06249999999999645, 2.071067811865478614 ) ) ;
#9838=CARTESIAN_POINT ( 'NONE',  ( 1.846868145590736310, -25.62500000136559564, 4.458734124999999437 ) ) ;
#9841=ORIENTED_EDGE ( 'NONE', *, *, #14088, .F. ) ;
#9846=CARTESIAN_POINT ( 'NONE',  ( 2.730187237215162345E-16, -23.18750000136559564, -4.458734124999999437 ) ) ;
#9848=EDGE_LOOP ( 'NONE', ( #11824, #5051, #3887, #7801, #11843 ) ) ;
#9850=VECTOR ( 'NONE', #517, 1000.000000000000000 ) ;
#9851=CARTESIAN_POINT ( 'NONE',  ( 0.000000000000000000, -20.00000000000000000, 0.000000000000000000 ) ) ;
#9856=CARTESIAN_POINT ( 'NONE',  ( 4.458734125000000326, -24.62500000136559564, -1.846868145590734978 ) ) ;
#9859=CARTESIAN_POINT ( 'NONE',  ( 5.000000000000000000, -29.18750000273119127, 2.071067811865478614 ) ) ;
#9861=CARTESIAN_POINT ( 'NONE',  ( 3.535533905932736864, -24.25000000273118772, 3.535533905932738641 ) ) ;
#9867=DIRECTION ( 'NONE',  ( 0.000000000000000000, 1.000000000000000000, 0.000000000000000000 ) ) ;
#9873=CIRCLE ( 'NONE', #13215, 2.649999999999985700 ) ;
#9883=ORIENTED_EDGE ( 'NONE', *, *, #8811, .T. ) ;
#9888=CARTESIAN_POINT ( 'NONE',  ( 0.000000000000000000, -11.00000000000000178, 0.000000000000000000 ) ) ;
#9890=CARTESIAN_POINT ( 'NONE',  ( -2.071067811865469288, -30.43750000273118772, 5.000000000000007994 ) ) ;
#9894=CARTESIAN_POINT ( 'NONE',  ( 1.846868145590736310, -26.87500000136559919, 4.458734124999997661 ) ) ;
#9895=CARTESIAN_POINT ( 'NONE',  ( 3.152801135295366208, -22.56250000136559564, 3.152801135295367985 ) ) ;
#9897=LINE ( 'NONE', #14836, #5831 ) ;
#9898=ORIENTED_EDGE ( 'NONE', *, *, #846, .F. ) ;
#9902=CARTESIAN_POINT ( 'NONE',  ( 3.535533905932738197, -31.00000000273118772, -3.535533905932738197 ) ) ;
#9913=CARTESIAN_POINT ( 'NONE',  ( 3.152801135295367541, -27.31250000136559564, -3.152801135295367541 ) ) ;
#9918=ORIENTED_EDGE ( 'NONE', *, *, #12068, .T. ) ;
#9922=CARTESIAN_POINT ( 'NONE',  ( 4.458734125000000326, -24.37500000136559564, -1.846868145590734978 ) ) ;
#9923=ADVANCED_FACE ( 'NONE', ( #11459 ), #3873, .T. ) ;
#9931=( BOUNDED_CURVE ( )  B_SPLINE_CURVE ( 2, ( #4166, #4339, #1821, #2949, #11672, #627, #10481, #9347, #15414 ),
 .UNSPECIFIED., .F., .F. ) 
 B_SPLINE_CURVE_WITH_KNOTS ( ( 3, 2, 2, 2, 3 ),
 ( 0.4750000000000000888, 0.4875000000000000999, 0.5000000000000001110, 0.5125000000000000666, 0.5250000000000001332 ),
 .UNSPECIFIED. ) 
 CURVE ( )  GEOMETRIC_REPRESENTATION_ITEM ( )  RATIONAL_B_SPLINE_CURVE ( ( 0.9999999999999993339, 0.9238795325112874046, 1.000000000000000000, 0.9238795325112867385, 1.000000000000000000, 0.9238795325112867385, 1.000000000000000000, 0.9238795325112860723, 1.000000000000000666 ) ) 
 REPRESENTATION_ITEM ( '' )  );
#9932=CARTESIAN_POINT ( 'NONE',  ( 5.000000000000000888, -28.93750000000000355, -2.071067811865475505 ) ) ;
#9936=CARTESIAN_POINT ( 'NONE',  ( 3.061616997868383141E-16, -26.87500000273118772, -5.000000000000000000 ) ) ;
#9938=CARTESIAN_POINT ( 'NONE',  ( 6.123233995736766282E-16, -20.00000000000000000, -5.000000000000000000 ) ) ;
#9939=CARTESIAN_POINT ( 'NONE',  ( -4.458734124999999437, -31.00000000136559564, -1.846868145590735644 ) ) ;
#9943=ORIENTED_EDGE ( 'NONE', *, *, #11652, .T. ) ;
#9948=LINE ( 'NONE', #3356, #3516 ) ;
#9957=CARTESIAN_POINT ( 'NONE',  ( 5.000000000000000888, -23.93750000000000355, -2.071067811865475505 ) ) ;
#9971=VECTOR ( 'NONE', #15081, 1000.000000000000000 ) ;
#9973=DIRECTION ( 'NONE',  ( -0.8660254037844385966, -0.5000000000000001110, 0.000000000000000000 ) ) ;
#9979=CARTESIAN_POINT ( 'NONE',  ( 5.000000000000000000, -28.12500000273118772, 0.000000000000000000 ) ) ;
#9980=CARTESIAN_POINT ( 'NONE',  ( 4.458734124999997661, -27.75000000136559564, 1.846868145590737864 ) ) ;
#9984=LINE ( 'NONE', #1330, #15131 ) ;
#9995=CARTESIAN_POINT ( 'NONE',  ( 4.458734124999999437, -23.75000000136559208, 1.846868145590737864 ) ) ;
#10003=CARTESIAN_POINT ( 'NONE',  ( 3.152801135295366208, -25.56250000136559564, 3.152801135295367985 ) ) ;
#10007=CARTESIAN_POINT ( 'NONE',  ( 35.00000000000000000, 37.00000000000000000, -5.999999999999991118 ) ) ;
#10014=CARTESIAN_POINT ( 'NONE',  ( -3.152801135295367985, -24.81250000136559564, 3.152801135295367096 ) ) ;
#10021=AXIS2_PLACEMENT_3D ( 'NONE', #7087, #1017, #13433 ) ;
#10025=CARTESIAN_POINT ( 'NONE',  ( -5.000000000000000000, -30.50000000000000000, -6.123233995736766282E-16 ) ) ;
#10029=CARTESIAN_POINT ( 'NONE',  ( 3.061616997868383141E-16, -29.87500000273118417, -5.000000000000000000 ) ) ;
#10032=CARTESIAN_POINT ( 'NONE',  ( 1.846868145590735200, -30.25000000136559919, -4.458734124999999437 ) ) ;
#10038=VECTOR ( 'NONE', #936, 1000.000000000000000 ) ;
#10039=CIRCLE ( 'NONE', #11831, 5.000000000000000000 ) ;
#10042=VECTOR ( 'NONE', #6488, 1000.000000000000000 ) ;
#10044=CARTESIAN_POINT ( 'NONE',  ( -4.458734125000001214, -31.12500000136559564, 1.846868145590734089 ) ) ;
#10050=FACE_OUTER_BOUND ( 'NONE', #12900, .T. ) ;
#10051=ORIENTED_EDGE ( 'NONE', *, *, #9169, .T. ) ;
#10053=( LENGTH_UNIT ( ) NAMED_UNIT ( * ) SI_UNIT ( .MILLI., .METRE. ) );
#10054=EDGE_LOOP ( 'NONE', ( #7174, #10132, #15157, #2662 ) ) ;
#10070=CARTESIAN_POINT ( 'NONE',  ( 4.769696007084728073, -20.00000000000000000, -1.500000000000000000 ) ) ;
#10084=CARTESIAN_POINT ( 'NONE',  ( 3.535533905932738197, -25.87500000000000355, -3.535533905932738197 ) ) ;
#10089=CARTESIAN_POINT ( 'NONE',  ( 5.000000000000000888, -29.93750000000000355, -2.071067811865475505 ) ) ;
#10091=CARTESIAN_POINT ( 'NONE',  ( -3.152801135295367096, -25.06250000136559564, -3.152801135295367541 ) ) ;
#10093=VERTEX_POINT ( 'NONE', #661 ) ;
#10095=VERTEX_POINT ( 'NONE', #15604 ) ;
#10097=CARTESIAN_POINT ( 'NONE',  ( 4.458734124999999437, -21.43750000136559208, 0.000000000000000000 ) ) ;
#10104=CARTESIAN_POINT ( 'NONE',  ( 2.071067811865475505, -28.81250000000000355, -5.000000000000000888 ) ) ;
#10106=CARTESIAN_POINT ( 'NONE',  ( 35.00000000000000000, 37.00000000000000000, 5.999999999999991118 ) ) ;
#10107=CARTESIAN_POINT ( 'NONE',  ( 5.000000000000000000, -27.18750000273119127, 2.071067811865478614 ) ) ;
#10109=CARTESIAN_POINT ( 'NONE',  ( 5.000000000000000888, -24.06250000273118772, -2.071067811865475505 ) ) ;
#10112=ORIENTED_EDGE ( 'NONE', *, *, #9740, .T. ) ;
#10117=ORIENTED_EDGE ( 'NONE', *, *, #12499, .F. ) ;
#10126=VERTEX_POINT ( 'NONE', #1853 ) ;
#10132=ORIENTED_EDGE ( 'NONE', *, *, #8085, .T. ) ;
#10139=CARTESIAN_POINT ( 'NONE',  ( 3.535533905932736864, -21.25000000273118772, 3.535533905932738641 ) ) ;
#10142=CARTESIAN_POINT ( 'NONE',  ( -5.000000000000000000, -30.62500000273118772, -6.123233995736766282E-16 ) ) ;
#10144=CARTESIAN_POINT ( 'NONE',  ( -9.184850993605147944E-16, -23.25000000000000000, 5.000000000000000000 ) ) ;
#10146=CARTESIAN_POINT ( 'NONE',  ( 4.458734124999999437, -21.68750000136559208, 0.000000000000000000 ) ) ;
#10167=CARTESIAN_POINT ( 'NONE',  ( 4.458734125000000326, -22.37500000136559564, -1.846868145590734978 ) ) ;
#10174=CARTESIAN_POINT ( 'NONE',  ( -3.152801135295367096, -30.31250000136559564, -3.152801135295367541 ) ) ;
#10180=CARTESIAN_POINT ( 'NONE',  ( -5.000000000000000000, -28.50000000000000000, -6.123233995736766282E-16 ) ) ;
#10181=( BOUNDED_CURVE ( )  B_SPLINE_CURVE ( 2, ( #6060, #5820, #8503, #12181, #13313 ),
 .UNSPECIFIED., .F., .F. ) 
 B_SPLINE_CURVE_WITH_KNOTS ( ( 3, 2, 3 ),
 ( 0.9750000000000001998, 0.9875000000000001554, 1.000000000000000000 ),
 .UNSPECIFIED. ) 
 CURVE ( )  GEOMETRIC_REPRESENTATION_ITEM ( )  RATIONAL_B_SPLINE_CURVE ( ( 0.9999999999999986677, 0.9238795325112880708, 1.000000000000000000, 0.9238795325112867385, 1.000000000000000000 ) ) 
 REPRESENTATION_ITEM ( '' )  );
#10185=CARTESIAN_POINT ( 'NONE',  ( 2.071067811865475505, -30.81250000000000000, -5.000000000000000888 ) ) ;
#10188=CARTESIAN_POINT ( 'NONE',  ( -9.184850993605147944E-16, -24.37500000273118772, 5.000000000000000000 ) ) ;
#10191=CARTESIAN_POINT ( 'NONE',  ( -4.458734125000000326, -30.87500000136559564, 1.846868145590734089 ) ) ;
#10196=VERTEX_POINT ( 'NONE', #12837 ) ;
#10205=DIRECTION ( 'NONE',  ( 0.000000000000000000, -0.000000000000000000, 1.000000000000000000 ) ) ;
#10216=CARTESIAN_POINT ( 'NONE',  ( 4.458734125000000326, -31.37500000136559564, -1.846868145590734978 ) ) ;
#10217=ADVANCED_FACE ( 'NONE', ( #4841 ), #3388, .F. ) ;
#10221=FACE_BOUND ( 'NONE', #136, .T. ) ;
#10229=EDGE_CURVE ( 'NONE', #7272, #8967, #10749, .T. ) ;
#10231=CARTESIAN_POINT ( 'NONE',  ( -8.190561711645485556E-16, -22.93750000136559564, 4.458734124999999437 ) ) ;
#10237=VERTEX_POINT ( 'NONE', #13229 ) ;
#10238=COLOUR_RGB ( '', 0.08235294, 0.09019608, 0.10196078) ;
#10250=ADVANCED_FACE ( 'NONE', ( #4678 ), #15921, .T. ) ;
#10253=CARTESIAN_POINT ( 'NONE',  ( -3.152801135295367096, -24.06250000136559564, -3.152801135295367541 ) ) ;
#10258=PLANE ( 'NONE',  #12525 ) ;
#10261=ADVANCED_BREP_SHAPE_REPRESENTATION ( '', ( #9346, #3223 ), #15660 ) ;
#10263=CARTESIAN_POINT ( 'NONE',  ( -3.152801135295367985, -30.06250000136559564, 3.152801135295367096 ) ) ;
#10271=CARTESIAN_POINT ( 'NONE',  ( 5.000000000000000000, -30.06250000000000000, 2.071067811865478614 ) ) ;
#10276=CARTESIAN_POINT ( 'NONE',  ( 5.000000000000000888, -24.06250000273118417, -2.071067811865475505 ) ) ;
#10278=CARTESIAN_POINT ( 'NONE',  ( 2.730187237215162345E-16, -26.18750000136559564, -4.458734124999999437 ) ) ;
#10291=CARTESIAN_POINT ( 'NONE',  ( -4.458734124999999437, -30.18750000136559564, -5.460374474430324690E-16 ) ) ;
#10296=ADVANCED_FACE ( 'NONE', ( #9680 ), #14618, .T. ) ;
#10304=CARTESIAN_POINT ( 'NONE',  ( -3.152801135295367985, -30.81250000136559564, 3.152801135295367096 ) ) ;
#10311=CARTESIAN_POINT ( 'NONE',  ( -5.000000000000000000, -28.62500000273118772, -6.123233995736766282E-16 ) ) ;
#10317=CARTESIAN_POINT ( 'NONE',  ( 4.458734124999999437, -22.68750000136559564, 0.000000000000000000 ) ) ;
#10323=LINE ( 'NONE', #13710, #14179 ) ;
#10326=AXIS2_PLACEMENT_3D ( 'NONE', #9324, #2037, #7293 ) ;
#10336=CARTESIAN_POINT ( 'NONE',  ( -8.190561711645485556E-16, -22.68750000136559564, 4.458734124999999437 ) ) ;
#10338=ORIENTED_EDGE ( 'NONE', *, *, #14054, .F. ) ;
#10341=ORIENTED_EDGE ( 'NONE', *, *, #3148, .T. ) ;
#10342=CARTESIAN_POINT ( 'NONE',  ( 4.458734124999999437, -22.50000000136559208, 1.846868145590737864 ) ) ;
#10350=CARTESIAN_POINT ( 'NONE',  ( 2.071067811865475505, -27.81250000000000000, -5.000000000000000888 ) ) ;
#10354=CARTESIAN_POINT ( 'NONE',  ( 5.000000000000000000, -26.18750000273119127, 2.071067811865478614 ) ) ;
#10355=LINE ( 'NONE', #2982, #10672 ) ;
#10356=CARTESIAN_POINT ( 'NONE',  ( -4.458734124999999437, -25.00000000136559564, -1.846868145590735644 ) ) ;
#10359=ORIENTED_EDGE ( 'NONE', *, *, #6446, .F. ) ;
#10363=CARTESIAN_POINT ( 'NONE',  ( -35.00000000000000000, 37.00000000000000000, 0.000000000000000000 ) ) ;
#10367=CARTESIAN_POINT ( 'NONE',  ( -8.190561711645485556E-16, -30.93750000136559564, 4.458734124999999437 ) ) ;
#10368=CARTESIAN_POINT ( 'NONE',  ( 0.000000000000000000, 20.00000000000000000, 5.000000000000000000 ) ) ;
#10377=CARTESIAN_POINT ( 'NONE',  ( -1.846868145590737420, -28.75000000136559208, 4.458734124999999437 ) ) ;
#10378=VERTEX_POINT ( 'NONE', #6593 ) ;
#10379=EDGE_CURVE ( 'NONE', #6271, #13973, #10323, .T. ) ;
#10382=VECTOR ( 'NONE', #822, 1000.000000000000000 ) ;
#10401=CARTESIAN_POINT ( 'NONE',  ( 0.000000000000000000, -20.00000000000000000, 0.000000000000000000 ) ) ;
#10402=AXIS2_PLACEMENT_3D ( 'NONE', #9078, #15375, #15051 ) ;
#10405=CARTESIAN_POINT ( 'NONE',  ( -1.846868145590734756, -23.12500000136559564, -4.458734125000000326 ) ) ;
#10412=CARTESIAN_POINT ( 'NONE',  ( -3.152801135295367985, -21.81250000136559208, 3.152801135295367096 ) ) ;
#10420=CARTESIAN_POINT ( 'NONE',  ( -35.00000000000000000, 37.00000000000000000, 2.649999999999992806 ) ) ;
#10421=CARTESIAN_POINT ( 'NONE',  ( -2.071067811865478170, -25.31250000000000000, 5.000000000000000000 ) ) ;
#10425=CARTESIAN_POINT ( 'NONE',  ( -9.184850993605147944E-16, -26.37500000273118417, 5.000000000000000000 ) ) ;
#10427=CARTESIAN_POINT ( 'NONE',  ( -4.458734124999999437, -27.00000000136559564, -1.846868145590735644 ) ) ;
#10434=EDGE_LOOP ( 'NONE', ( #7616, #8964, #7158, #7533 ) ) ;
#10439=CARTESIAN_POINT ( 'NONE',  ( -3.152801135295367985, -29.06250000136559564, 3.152801135295367096 ) ) ;
#10442=CARTESIAN_POINT ( 'NONE',  ( -24.26932219902320043, 37.00000000000000000, 5.999999999999998224 ) ) ;
#10457=DIRECTION ( 'NONE',  ( 0.000000000000000000, 0.000000000000000000, 1.000000000000000000 ) ) ;
#10465=EDGE_CURVE ( 'NONE', #7938, #6661, #9416, .T. ) ;
#10470=CARTESIAN_POINT ( 'NONE',  ( -5.000000000000000000, -26.62500000273118772, -6.123233995736766282E-16 ) ) ;
#10474=ORIENTED_EDGE ( 'NONE', *, *, #8019, .F. ) ;
#10475=CARTESIAN_POINT ( 'NONE',  ( -9.184850993605147944E-16, -30.25000000000000000, 5.000000000000000000 ) ) ;
#10476=DIRECTION ( 'NONE',  ( -0.000000000000000000, 1.000000000000000000, -0.000000000000000000 ) ) ;
#10478=FACE_OUTER_BOUND ( 'NONE', #6557, .T. ) ;
#10480=VECTOR ( 'NONE', #8573, 1000.000000000000000 ) ;
#10481=CARTESIAN_POINT ( 'NONE',  ( 3.535533905932738197, -26.00000000273118417, -3.535533905932738197 ) ) ;
#10489=CARTESIAN_POINT ( 'NONE',  ( 1.846868145590736310, -24.62500000136559564, 4.458734124999999437 ) ) ;
#10500=CARTESIAN_POINT ( 'NONE',  ( 3.152801135295367541, -25.56250000136559564, -3.152801135295367541 ) ) ;
#10509=CARTESIAN_POINT ( 'NONE',  ( -5.000000000000000888, -24.43750000000000355, 2.071067811865474617 ) ) ;
#10514=CARTESIAN_POINT ( 'NONE',  ( -5.000000000000000000, -24.62500000273118417, -6.123233995736766282E-16 ) ) ;
#10517=CARTESIAN_POINT ( 'NONE',  ( 4.458734124999997661, -24.50000000136559564, 1.846868145590737864 ) ) ;
#10522=CARTESIAN_POINT ( 'NONE',  ( 0.000000000000000000, -20.00000000000000000, 0.000000000000000000 ) ) ;
#10524=ORIENTED_EDGE ( 'NONE', *, *, #4976, .F. ) ;
#10528=CARTESIAN_POINT ( 'NONE',  ( 2.730187237215162345E-16, -28.43750000136559564, -4.458734124999999437 ) ) ;
#10537=ORIENTED_EDGE ( 'NONE', *, *, #14054, .T. ) ;
#10550=AXIS2_PLACEMENT_3D ( 'NONE', #3729, #1472, #8764 ) ;
#10557=CARTESIAN_POINT ( 'NONE',  ( -35.00000000000000000, 37.00000000000000000, 0.000000000000000000 ) ) ;
#10561=VERTEX_POINT ( 'NONE', #14426 ) ;
#10564=VERTEX_POINT ( 'NONE', #9568 ) ;
#10574=CARTESIAN_POINT ( 'NONE',  ( -3.535533905932738641, -25.37500000000000000, 3.535533905932737309 ) ) ;
#10579=CARTESIAN_POINT ( 'NONE',  ( -4.458734124999999437, -28.18750000136559564, -5.460374474430324690E-16 ) ) ;
#10585=ORIENTED_EDGE ( 'NONE', *, *, #14247, .F. ) ;
#10586=CARTESIAN_POINT ( 'NONE',  ( -8.190561711645485556E-16, -27.93750000136559564, 4.458734124999999437 ) ) ;
#10589=CYLINDRICAL_SURFACE ( 'NONE', #12267, 5.000000000000000000 ) ;
#10590=EDGE_CURVE ( 'NONE', #14037, #8368, #880, .T. ) ;
#10595=CARTESIAN_POINT ( 'NONE',  ( 3.535533905932738197, -27.87500000000000000, -3.535533905932738197 ) ) ;
#10599=CARTESIAN_POINT ( 'NONE',  ( 5.000000000000000000, -22.18750000273118772, 2.071067811865478614 ) ) ;
#10601=CARTESIAN_POINT ( 'NONE',  ( -4.458734124999999437, -22.00000000136559208, -1.846868145590735644 ) ) ;
#10610=CARTESIAN_POINT ( 'NONE',  ( 4.458734124999999437, -28.75000000136559208, 1.846868145590737864 ) ) ;
#10611=DIRECTION ( 'NONE',  ( 0.000000000000000000, 1.000000000000000000, 0.000000000000000000 ) ) ;
#10619=VERTEX_POINT ( 'NONE', #14737 ) ;
#10622=CARTESIAN_POINT ( 'NONE',  ( -9.184850993605147944E-16, -28.25000000000000000, 5.000000000000000000 ) ) ;
#10630=CARTESIAN_POINT ( 'NONE',  ( 5.000000000000000000, -21.12500000273118772, 0.000000000000000000 ) ) ;
#10633=CARTESIAN_POINT ( 'NONE',  ( 3.535533905932738197, -26.87500000000000000, -3.535533905932738197 ) ) ;
#10634=ORIENTED_EDGE ( 'NONE', *, *, #13397, .F. ) ;
#10637=FACE_OUTER_BOUND ( 'NONE', #11659, .T. ) ;
#10639=CARTESIAN_POINT ( 'NONE',  ( 3.061616997868383141E-16, -22.87500000273118772, -5.000000000000000000 ) ) ;
#10654=CARTESIAN_POINT ( 'NONE',  ( -4.458734125000001214, -26.12500000136559919, 1.846868145590734089 ) ) ;
#10655=DIRECTION ( 'NONE',  ( -0.000000000000000000, 1.000000000000000000, -0.000000000000000000 ) ) ;
#10659=CARTESIAN_POINT ( 'NONE',  ( -5.000000000000000888, -27.43750000000000711, 2.071067811865474617 ) ) ;
#10663=CARTESIAN_POINT ( 'NONE',  ( 3.061616997868383141E-16, -21.87500000273118772, -5.000000000000000000 ) ) ;
#10665=CARTESIAN_POINT ( 'NONE',  ( -4.458734125000000326, -22.87500000136559564, 1.846868145590734089 ) ) ;
#10672=VECTOR ( 'NONE', #2740, 1000.000000000000114 ) ;
#10673=CARTESIAN_POINT ( 'NONE',  ( -1.846868145590734756, -28.12500000136559564, -4.458734125000000326 ) ) ;
#10680=CARTESIAN_POINT ( 'NONE',  ( -1.846868145590737420, -29.00000000136559564, 4.458734124999999437 ) ) ;
#10687=EDGE_LOOP ( 'NONE', ( #15836, #10727, #15366, #4941 ) ) ;
#10689=ORIENTED_EDGE ( 'NONE', *, *, #713, .T. ) ;
#10692=( BOUNDED_CURVE ( )  B_SPLINE_CURVE ( 2, ( #62, #9662, #3521, #3683, #6039, #7417, #13289, #13376, #9590 ),
 .UNSPECIFIED., .F., .F. ) 
 B_SPLINE_CURVE_WITH_KNOTS ( ( 3, 2, 2, 2, 3 ),
 ( 0.07500000000000006661, 0.08750000000000007772, 0.1000000000000000888, 0.1125000000000000999, 0.1250000000000001110 ),
 .UNSPECIFIED. ) 
 CURVE ( )  GEOMETRIC_REPRESENTATION_ITEM ( )  RATIONAL_B_SPLINE_CURVE ( ( 0.9999999999999995559, 0.9238795325112871826, 1.000000000000000000, 0.9238795325112867385, 1.000000000000000000, 0.9238795325112867385, 1.000000000000000000, 0.9238795325112860723, 1.000000000000000666 ) ) 
 REPRESENTATION_ITEM ( '' )  );
#10700=EDGE_LOOP ( 'NONE', ( #4463, #2788, #8471, #9123 ) ) ;
#10707=ORIENTED_EDGE ( 'NONE', *, *, #6935, .T. ) ;
#10709=EDGE_LOOP ( 'NONE', ( #6574, #4102 ) ) ;
#10722=CARTESIAN_POINT ( 'NONE',  ( 3.152801135295367541, -30.56250000136559564, -3.152801135295367541 ) ) ;
#10727=ORIENTED_EDGE ( 'NONE', *, *, #14729, .F. ) ;
#10729=CARTESIAN_POINT ( 'NONE',  ( 2.730187237215162345E-16, -27.43750000136559564, -4.458734124999999437 ) ) ;
#10737=CARTESIAN_POINT ( 'NONE',  ( -2.071067811865475061, -22.68749999999999645, -5.000000000000000888 ) ) ;
#10740=CARTESIAN_POINT ( 'NONE',  ( -5.000000000000000888, -21.68750000273119127, -2.071067811865475949 ) ) ;
#10742=CARTESIAN_POINT ( 'NONE',  ( -4.458734124999999437, -28.93750000136559564, -5.460374474430324690E-16 ) ) ;
#10743=CIRCLE ( 'NONE', #7395, 5.000000000000000000 ) ;
#10745=CARTESIAN_POINT ( 'NONE',  ( -1.846868145590737420, -21.75000000136559208, 4.458734124999997661 ) ) ;
#10749=LINE ( 'NONE', #14465, #1786 ) ;
#10750=CARTESIAN_POINT ( 'NONE',  ( -4.458734125000000326, -29.00000000136559564, -1.846868145590735644 ) ) ;
#10752=EDGE_LOOP ( 'NONE', ( #2015, #14617, #93, #10825, #12231, #8866, #6318, #1993 ) ) ;
#10760=CARTESIAN_POINT ( 'NONE',  ( 3.152801135295367541, -29.56250000136559208, -3.152801135295367541 ) ) ;
#10785=ORIENTED_EDGE ( 'NONE', *, *, #4507, .F. ) ;
#10790=CARTESIAN_POINT ( 'NONE',  ( 3.061616997868383141E-16, -30.75000000000000000, -5.000000000000000000 ) ) ;
#10792=DIRECTION ( 'NONE',  ( 0.000000000000000000, 0.000000000000000000, -1.000000000000000000 ) ) ;
#10796=CYLINDRICAL_SURFACE ( 'NONE', #5604, 25.00000000000000000 ) ;
#10802=CARTESIAN_POINT ( 'NONE',  ( -3.152801135295367985, -30.06250000136559564, 3.152801135295367096 ) ) ;
#10807=AXIS2_PLACEMENT_3D ( 'NONE', #3669, #6739, #12462 ) ;
#10810=ORIENTED_EDGE ( 'NONE', *, *, #14209, .F. ) ;
#10811=CARTESIAN_POINT ( 'NONE',  ( -4.458734124999999437, -26.18750000136559919, -5.460374474430324690E-16 ) ) ;
#10822=CARTESIAN_POINT ( 'NONE',  ( -3.535533905932737309, -21.75000000273118772, -3.535533905932738197 ) ) ;
#10825=ORIENTED_EDGE ( 'NONE', *, *, #601, .T. ) ;
#10827=CARTESIAN_POINT ( 'NONE',  ( 3.152801135295366208, -29.56250000136559208, 3.152801135295367985 ) ) ;
#10829=DIRECTION ( 'NONE',  ( 0.000000000000000000, 1.000000000000000000, 0.000000000000000000 ) ) ;
#10836=CARTESIAN_POINT ( 'NONE',  ( -4.458734125000000326, -23.25000000136559208, -1.846868145590735644 ) ) ;
#10844=DIRECTION ( 'NONE',  ( 0.000000000000000000, 1.000000000000000000, 0.000000000000000000 ) ) ;
#10848=CARTESIAN_POINT ( 'NONE',  ( -9.184850993605147944E-16, -25.37500000273118417, 5.000000000000000000 ) ) ;
#10871=CARTESIAN_POINT ( 'NONE',  ( 3.152801135295367541, -27.56250000136559564, -3.152801135295367541 ) ) ;
#10881=CARTESIAN_POINT ( 'NONE',  ( 3.152801135295367541, -22.56250000136559564, -3.152801135295367541 ) ) ;
#10887=CARTESIAN_POINT ( 'NONE',  ( 3.535533905932736864, -23.12500000000000000, 3.535533905932738641 ) ) ;
#10891=CARTESIAN_POINT ( 'NONE',  ( -3.535533905932738641, -21.50000000273118772, 3.535533905932737309 ) ) ;
#10897=ORIENTED_EDGE ( 'NONE', *, *, #1043, .F. ) ;
#10900=CARTESIAN_POINT ( 'NONE',  ( 1.846868145590735200, -27.25000000136559564, -4.458734125000000326 ) ) ;
#10904=CARTESIAN_POINT ( 'NONE',  ( 0.000000000000000000, 20.00000000000000000, 0.000000000000000000 ) ) ;
#10908=CARTESIAN_POINT ( 'NONE',  ( -4.458734124999999437, -22.18750000136559564, -5.460374474430324690E-16 ) ) ;
#10915=CARTESIAN_POINT ( 'NONE',  ( 0.000000000000000000, -13.00000000000000178, 0.000000000000000000 ) ) ;
#10916=CARTESIAN_POINT ( 'NONE',  ( 3.535533905932736864, -25.12500000000000000, 3.535533905932738641 ) ) ;
#10922=CARTESIAN_POINT ( 'NONE',  ( -2.071067811865492381, -26.31250000000000355, 4.999999999999985789 ) ) ;
#10928=PRODUCT_DEFINITION_SHAPE ( 'NONE', 'NONE',  #11724 ) ;
#10933=ORIENTED_EDGE ( 'NONE', *, *, #2261, .F. ) ;
#10943=DIRECTION ( 'NONE',  ( 0.000000000000000000, 0.000000000000000000, 1.000000000000000000 ) ) ;
#10950=CARTESIAN_POINT ( 'NONE',  ( -1.846868145590734756, -25.37500000136559564, -4.458734124999999437 ) ) ;
#10957=CARTESIAN_POINT ( 'NONE',  ( -4.458734125000000326, -23.25000000136559208, -1.846868145590735644 ) ) ;
#10965=EDGE_CURVE ( 'NONE', #9262, #10093, #1266, .T. ) ;
#10969=CARTESIAN_POINT ( 'NONE',  ( 0.000000000000000000, -20.00000000000000000, 5.000000000000000000 ) ) ;
#10970=CARTESIAN_POINT ( 'NONE',  ( 0.000000000000000000, -20.00000000000000000, 1.500000000000000000 ) ) ;
#10971=CARTESIAN_POINT ( 'NONE',  ( -3.152801135295367985, -27.81250000136559564, 3.152801135295367096 ) ) ;
#10973=( BOUNDED_CURVE ( )  B_SPLINE_CURVE ( 2, ( #2955, #2634, #7759, #240, #6372, #10089, #8875, #5159, #7829 ),
 .UNSPECIFIED., .F., .F. ) 
 B_SPLINE_CURVE_WITH_KNOTS ( ( 3, 2, 2, 2, 3 ),
 ( 0.1750000000000001554, 0.1875000000000001665, 0.2000000000000001776, 0.2125000000000001887, 0.2250000000000001998 ),
 .UNSPECIFIED. ) 
 CURVE ( )  GEOMETRIC_REPRESENTATION_ITEM ( )  RATIONAL_B_SPLINE_CURVE ( ( 0.9999999999999990008, 0.9238795325112877377, 1.000000000000000000, 0.9238795325112867385, 1.000000000000000000, 0.9238795325112867385, 1.000000000000000000, 0.9238795325112855172, 1.000000000000001110 ) ) 
 REPRESENTATION_ITEM ( '' )  );
#10982=CARTESIAN_POINT ( 'NONE',  ( 4.458734124999999437, -23.50000000136559564, 1.846868145590737864 ) ) ;
#10985=CARTESIAN_POINT ( 'NONE',  ( 0.000000000000000000, -20.00000000000000000, 5.000000000000000000 ) ) ;
#10992=CARTESIAN_POINT ( 'NONE',  ( 4.458734125000000326, -23.62500000136559919, -1.846868145590734978 ) ) ;
#10996=CARTESIAN_POINT ( 'NONE',  ( -2.071067811865478170, -27.43750000273119127, 5.000000000000000000 ) ) ;
#11027=CARTESIAN_POINT ( 'NONE',  ( 4.458734124999999437, -22.43750000136559564, 0.000000000000000000 ) ) ;
#11028=DIRECTION ( 'NONE',  ( 0.000000000000000000, 1.000000000000000000, 0.000000000000000000 ) ) ;
#11030=DIRECTION ( 'NONE',  ( -1.000000000000000000, 0.000000000000000000, 1.239088197126290570E-16 ) ) ;
#11033=DIRECTION ( 'NONE',  ( 0.000000000000000000, 0.000000000000000000, 1.000000000000000000 ) ) ;
#11035=CARTESIAN_POINT ( 'NONE',  ( -2.071067811865489272, -22.81250000273118417, -4.999999999999985789 ) ) ;
#11036=CARTESIAN_POINT ( 'NONE',  ( -3.152801135295367096, -24.31250000136559564, -3.152801135295367541 ) ) ;
#11037=CARTESIAN_POINT ( 'NONE',  ( 1.846868145590736310, -22.62500000136559564, 4.458734124999997661 ) ) ;
#11045=CARTESIAN_POINT ( 'NONE',  ( 2.730187237215162345E-16, -24.43750000136559564, -4.458734124999999437 ) ) ;
#11047=CARTESIAN_POINT ( 'NONE',  ( -9.184850993605147944E-16, -23.37500000273118772, 5.000000000000000000 ) ) ;
#11049=CARTESIAN_POINT ( 'NONE',  ( -3.535533905932737309, -27.75000000273118772, -3.535533905932738197 ) ) ;
#11058=CARTESIAN_POINT ( 'NONE',  ( -3.535533905932738641, -27.37500000000000000, 3.535533905932737309 ) ) ;
#11059=CARTESIAN_POINT ( 'NONE',  ( 2.730187237215162345E-16, -27.18750000136559564, -4.458734124999999437 ) ) ;
#11064=VERTEX_POINT ( 'NONE', #6073 ) ;
#11067=CARTESIAN_POINT ( 'NONE',  ( 1.846868145590735200, -26.25000000136559208, -4.458734125000000326 ) ) ;
#11079=CARTESIAN_POINT ( 'NONE',  ( -3.152801135295367096, -22.31250000136559564, -3.152801135295367541 ) ) ;
#11082=CARTESIAN_POINT ( 'NONE',  ( -2.071067811865475061, -28.81250000273118772, -5.000000000000000888 ) ) ;
#11084=CARTESIAN_POINT ( 'NONE',  ( -3.152801135295367096, -30.06250000136559564, -3.152801135295367541 ) ) ;
#11092=CARTESIAN_POINT ( 'NONE',  ( -2.071067811865489272, -25.81250000273118417, -4.999999999999985789 ) ) ;
#11102=EDGE_CURVE ( 'NONE', #9435, #7272, #14350, .T. ) ;
#11113=CARTESIAN_POINT ( 'NONE',  ( -4.458734125000000326, -26.12500000136559919, 1.846868145590734089 ) ) ;
#11114=CARTESIAN_POINT ( 'NONE',  ( 3.152801135295366208, -21.56250000136559208, 3.152801135295367985 ) ) ;
#11121=CARTESIAN_POINT ( 'NONE',  ( 4.458734125000000326, -23.62500000136559919, -1.846868145590734978 ) ) ;
#11124=LINE ( 'NONE', #4668, #14516 ) ;
#11130=ADVANCED_FACE ( 'NONE', ( #2271 ), #7222, .T. ) ;
#11131=CARTESIAN_POINT ( 'NONE',  ( 2.730187237215162345E-16, -25.18750000136559564, -4.458734124999999437 ) ) ;
#11135=ORIENTED_EDGE ( 'NONE', *, *, #14466, .T. ) ;
#11138=CARTESIAN_POINT ( 'NONE',  ( 4.458734124999999437, -26.43750000136559564, 0.000000000000000000 ) ) ;
#11145=CARTESIAN_POINT ( 'NONE',  ( 5.000000000000000000, -31.06250000000000000, 2.071067811865478614 ) ) ;
#11150=CARTESIAN_POINT ( 'NONE',  ( -5.000000000000000888, -27.56250000273118772, 2.071067811865474617 ) ) ;
#11152=CARTESIAN_POINT ( 'NONE',  ( -1.846868145590737420, -28.75000000136559564, 4.458734124999997661 ) ) ;
#11159=CARTESIAN_POINT ( 'NONE',  ( -3.535533905932737309, -25.75000000273118417, -3.535533905932738197 ) ) ;
#11172=DIRECTION ( 'NONE',  ( 0.000000000000000000, 0.000000000000000000, -1.000000000000000000 ) ) ;
#11180=CARTESIAN_POINT ( 'NONE',  ( 3.535533905932738197, -27.00000000273118772, -3.535533905932738197 ) ) ;
#11184=CARTESIAN_POINT ( 'NONE',  ( 1.846868145590736310, -23.87500000136559564, 4.458734124999997661 ) ) ;
#11185=CIRCLE ( 'NONE', #4224, 2.649999999999992806 ) ;
#11194=CARTESIAN_POINT ( 'NONE',  ( 4.458734124999999437, -24.68750000136559564, 0.000000000000000000 ) ) ;
#11197=FACE_OUTER_BOUND ( 'NONE', #7594, .T. ) ;
#11202=( BOUNDED_CURVE ( )  B_SPLINE_CURVE ( 2, ( #3617, #6530, #11444, #5160, #7760, #11207, #2636, #1591, #7587 ),
 .UNSPECIFIED., .F., .F. ) 
 B_SPLINE_CURVE_WITH_KNOTS ( ( 3, 2, 2, 2, 3 ),
 ( 0.2749999999999999112, 0.2874999999999998668, 0.2999999999999999334, 0.3124999999999999445, 0.3249999999999999556 ),
 .UNSPECIFIED. ) 
 CURVE ( )  GEOMETRIC_REPRESENTATION_ITEM ( )  RATIONAL_B_SPLINE_CURVE ( ( 1.000000000000000666, 0.9238795325112860723, 1.000000000000000000, 0.9238795325112867385, 1.000000000000000000, 0.9238795325112867385, 1.000000000000000000, 0.9238795325112870716, 0.9999999999999996669 ) ) 
 REPRESENTATION_ITEM ( '' )  );
#11207=CARTESIAN_POINT ( 'NONE',  ( 5.000000000000000888, -28.93750000000000355, -2.071067811865475505 ) ) ;
#11208=CARTESIAN_POINT ( 'NONE',  ( 1.846868145590735200, -26.25000000136559208, -4.458734125000000326 ) ) ;
#11216=CARTESIAN_POINT ( 'NONE',  ( -4.458734125000000326, -26.00000000136559208, -1.846868145590735644 ) ) ;
#11226=CIRCLE ( 'NONE', #943, 5.000000000000000000 ) ;
#11227=CARTESIAN_POINT ( 'NONE',  ( 5.000000000000000000, -31.00000000000000000, 0.000000000000000000 ) ) ;
#11230=CARTESIAN_POINT ( 'NONE',  ( 3.535533905932736864, -29.25000000273118772, 3.535533905932738641 ) ) ;
#11240=DIRECTION ( 'NONE',  ( 0.000000000000000000, 0.000000000000000000, 1.000000000000000000 ) ) ;
#11242=VECTOR ( 'NONE', #4760, 1000.000000000000000 ) ;
#11244=CARTESIAN_POINT ( 'NONE',  ( -1.846868145590734756, -31.37500000136559564, -4.458734125000000326 ) ) ;
#11251=ORIENTED_EDGE ( 'NONE', *, *, #14488, .F. ) ;
#11256=DIRECTION ( 'NONE',  ( 0.000000000000000000, 0.000000000000000000, 1.000000000000000000 ) ) ;
#11270=CARTESIAN_POINT ( 'NONE',  ( 2.730187237215162345E-16, -23.43750000136559564, -4.458734124999999437 ) ) ;
#11284=DIRECTION ( 'NONE',  ( 0.000000000000000000, 0.000000000000000000, 1.000000000000000000 ) ) ;
#11292=CARTESIAN_POINT ( 'NONE',  ( -1.846868145590737420, -28.75000000136559208, 4.458734124999999437 ) ) ;
#11297=EDGE_LOOP ( 'NONE', ( #15703, #10341, #10785 ) ) ;
#11300=CARTESIAN_POINT ( 'NONE',  ( 1.846868145590736310, -24.62500000136559564, 4.458734124999999437 ) ) ;
#11301=CARTESIAN_POINT ( 'NONE',  ( 0.000000000000000000, -13.00000000000000178, -6.000000000000000888 ) ) ;
#11309=MECHANICAL_DESIGN_GEOMETRIC_PRESENTATION_REPRESENTATION('',(#7720),#2523);
#11310=CARTESIAN_POINT ( 'NONE',  ( -5.000000000000000888, -31.43750000000000355, 2.071067811865474617 ) ) ;
#11313=CARTESIAN_POINT ( 'NONE',  ( -5.000000000000000000, -28.62500000273118772, -6.123233995736766282E-16 ) ) ;
#11315=CARTESIAN_POINT ( 'NONE',  ( 3.152801135295366208, -30.56250000136559564, 3.152801135295367985 ) ) ;
#11325=DIRECTION ( 'NONE',  ( 0.000000000000000000, 0.000000000000000000, -1.000000000000000000 ) ) ;
#11327=CARTESIAN_POINT ( 'NONE',  ( 0.000000000000000000, 37.00000000000000000, 0.000000000000000000 ) ) ;
#11335=ORIENTED_EDGE ( 'NONE', *, *, #7794, .T. ) ;
#11340=DIRECTION ( 'NONE',  ( 0.000000000000000000, 1.000000000000000000, 0.000000000000000000 ) ) ;
#11351=FACE_OUTER_BOUND ( 'NONE', #689, .T. ) ;
#11362=CARTESIAN_POINT ( 'NONE',  ( -9.184850993605147944E-16, -27.37500000273118772, 5.000000000000000000 ) ) ;
#11368=EDGE_CURVE ( 'NONE', #580, #10196, #278, .T. ) ;
#11370=CARTESIAN_POINT ( 'NONE',  ( -1.846868145590737420, -23.75000000136559208, 4.458734124999999437 ) ) ;
#11373=ORIENTED_EDGE ( 'NONE', *, *, #12452, .F. ) ;
#11377=CARTESIAN_POINT ( 'NONE',  ( 1.846868145590735200, -29.50000000136559564, -4.458734125000000326 ) ) ;
#11380=CARTESIAN_POINT ( 'NONE',  ( -3.535533905932737309, -28.62500000000000000, -3.535533905932738197 ) ) ;
#11384=CARTESIAN_POINT ( 'NONE',  ( 3.535533905932736864, -30.12500000000000000, 3.535533905932738641 ) ) ;
#11387=CARTESIAN_POINT ( 'NONE',  ( 2.071067811865476394, -24.31250000273118772, 5.000000000000000000 ) ) ;
#11390=CARTESIAN_POINT ( 'NONE',  ( -1.846868145590737420, -30.75000000136559919, 4.458734124999997661 ) ) ;
#11402=DIRECTION ( 'NONE',  ( 0.000000000000000000, 1.000000000000000000, 0.000000000000000000 ) ) ;
#11411=CARTESIAN_POINT ( 'NONE',  ( -3.152801135295367096, -31.06250000136559564, -3.152801135295367541 ) ) ;
#11416=ADVANCED_FACE ( 'NONE', ( #14392 ), #3320, .T. ) ;
#11418=EDGE_CURVE ( 'NONE', #3993, #2783, #11707, .T. ) ;
#11425=CARTESIAN_POINT ( 'NONE',  ( 4.458734124999999437, -23.62500000136559564, -1.846868145590734978 ) ) ;
#11438=APPLICATION_CONTEXT ( 'automotive_design' ) ;
#11444=CARTESIAN_POINT ( 'NONE',  ( 3.535533905932736864, -29.12500000000000000, 3.535533905932738641 ) ) ;
#11445=CARTESIAN_POINT ( 'NONE',  ( 4.458734124999999437, -23.43750000136559564, 0.000000000000000000 ) ) ;
#11452=CARTESIAN_POINT ( 'NONE',  ( -4.458734124999999437, -21.93750000136559208, -5.460374474430324690E-16 ) ) ;
#11459=FACE_OUTER_BOUND ( 'NONE', #4390, .T. ) ;
#11462=CARTESIAN_POINT ( 'NONE',  ( -3.535533905932737309, -30.62500000000000000, -3.535533905932738197 ) ) ;
#11465=CARTESIAN_POINT ( 'NONE',  ( 3.061616997868383141E-16, -24.87500000273118417, -5.000000000000000000 ) ) ;
#11468=CARTESIAN_POINT ( 'NONE',  ( -3.152801135295367096, -27.06250000136559564, -3.152801135295367541 ) ) ;
#11477=EDGE_CURVE ( 'NONE', #8470, #12690, #2981, .T. ) ;
#11481=CARTESIAN_POINT ( 'NONE',  ( 4.458734125000000326, -31.62500000136559564, -1.846868145590734978 ) ) ;
#11484=PLANE ( 'NONE',  #7667 ) ;
#11495=AXIS2_PLACEMENT_3D ( 'NONE', #6031, #7253, #12153 ) ;
#11496=CARTESIAN_POINT ( 'NONE',  ( 3.061616997868383141E-16, -28.87500000273118772, -5.000000000000000000 ) ) ;
#11501=CARTESIAN_POINT ( 'NONE',  ( 3.152801135295366208, -21.81250000136559208, 3.152801135295367985 ) ) ;
#11505=CARTESIAN_POINT ( 'NONE',  ( -5.000000000000000888, -26.56250000273118772, 2.071067811865474617 ) ) ;
#11523=DIRECTION ( 'NONE',  ( 0.000000000000000000, 0.000000000000000000, 1.000000000000000000 ) ) ;
#11524=CARTESIAN_POINT ( 'NONE',  ( 4.458734124999997661, -26.75000000136559564, 1.846868145590737864 ) ) ;
#11533=CARTESIAN_POINT ( 'NONE',  ( -1.846868145590734756, -22.12500000136559564, -4.458734125000000326 ) ) ;
#11538=VECTOR ( 'NONE', #14108, 1000.000000000000000 ) ;
#11542=CARTESIAN_POINT ( 'NONE',  ( -5.000000000000000888, -26.56249999999999645, -2.071067811865475949 ) ) ;
#11547=CARTESIAN_POINT ( 'NONE',  ( -9.184850993605147944E-16, -30.37500000273118772, 5.000000000000000000 ) ) ;
#11548=CARTESIAN_POINT ( 'NONE',  ( 2.071067811865476394, -25.31250000273118062, 5.000000000000000000 ) ) ;
#11550=CARTESIAN_POINT ( 'NONE',  ( 3.152801135295367541, -27.31250000136559564, -3.152801135295367541 ) ) ;
#11562=CARTESIAN_POINT ( 'NONE',  ( 4.458734125000000326, -29.62500000136559208, -1.846868145590734978 ) ) ;
#11569=EDGE_LOOP ( 'NONE', ( #10933, #3994 ) ) ;
#11572=VERTEX_POINT ( 'NONE', #2331 ) ;
#11574=CARTESIAN_POINT ( 'NONE',  ( -3.152801135295367096, -30.06250000136559564, -3.152801135295367541 ) ) ;
#11582=( BOUNDED_CURVE ( )  B_SPLINE_CURVE ( 2, ( #293, #5206, #10139, #15065, #7734 ),
 .UNSPECIFIED., .F., .F. ) 
 B_SPLINE_CURVE_WITH_KNOTS ( ( 3, 2, 3 ),
 ( 0.9749999999999998668, 0.9875000000000000444, 1.000000000000000000 ),
 .UNSPECIFIED. ) 
 CURVE ( )  GEOMETRIC_REPRESENTATION_ITEM ( )  RATIONAL_B_SPLINE_CURVE ( ( 1.000000000000000666, 0.9238795325112860723, 1.000000000000000000, 0.9238795325112867385, 1.000000000000000000 ) ) 
 REPRESENTATION_ITEM ( '' )  );
#11586=CARTESIAN_POINT ( 'NONE',  ( -1.846868145590734756, -23.37500000136559564, -4.458734124999999437 ) ) ;
#11595=ORIENTED_EDGE ( 'NONE', *, *, #15753, .F. ) ;
#11603=CYLINDRICAL_SURFACE ( 'NONE', #11936, 5.000000000000000000 ) ;
#11604=CARTESIAN_POINT ( 'NONE',  ( 3.535533905932736864, -25.25000000273118417, 3.535533905932738641 ) ) ;
#11605=CARTESIAN_POINT ( 'NONE',  ( 1.846868145590736310, -21.62500000136559564, 4.458734124999999437 ) ) ;
#11611=CARTESIAN_POINT ( 'NONE',  ( -8.190561711645485556E-16, -21.68750000136559208, 4.458734124999999437 ) ) ;
#11612=DIRECTION ( 'NONE',  ( 0.000000000000000000, 1.000000000000000000, 0.000000000000000000 ) ) ;
#11620=CARTESIAN_POINT ( 'NONE',  ( 2.071067811865475505, -25.81250000000000000, -5.000000000000000888 ) ) ;
#11624=CARTESIAN_POINT ( 'NONE',  ( 2.071067811865475505, -23.93750000273119483, -5.000000000000000888 ) ) ;
#11626=CARTESIAN_POINT ( 'NONE',  ( -4.458734125000000326, -25.87500000136559564, 1.846868145590734089 ) ) ;
#11629=VERTEX_POINT ( 'NONE', #5325 ) ;
#11632=CARTESIAN_POINT ( 'NONE',  ( 5.000000000000000000, -29.18750000273119127, 2.071067811865478614 ) ) ;
#11633=ORIENTED_EDGE ( 'NONE', *, *, #3128, .F. ) ;
#11637=CARTESIAN_POINT ( 'NONE',  ( -4.458734125000001214, -28.12500000136559564, 1.846868145590734089 ) ) ;
#11652=EDGE_CURVE ( 'NONE', #2292, #13118, #8888, .T. ) ;
#11657=( LENGTH_UNIT ( ) NAMED_UNIT ( * ) SI_UNIT ( .MILLI., .METRE. ) );
#11659=EDGE_LOOP ( 'NONE', ( #4261, #12475, #7660, #5729 ) ) ;
#11663=ORIENTED_EDGE ( 'NONE', *, *, #521, .F. ) ;
#11665=ORIENTED_EDGE ( 'NONE', *, *, #4427, .T. ) ;
#11667=CARTESIAN_POINT ( 'NONE',  ( -2.071067811865489272, -30.68749999999999645, -4.999999999999985789 ) ) ;
#11668=FACE_OUTER_BOUND ( 'NONE', #15919, .T. ) ;
#11669=AXIS2_PLACEMENT_3D ( 'NONE', #8872, #15172, #4090 ) ;
#11670=CARTESIAN_POINT ( 'NONE',  ( 0.000000000000000000, -11.00000000000000178, 0.000000000000000000 ) ) ;
#11671=EDGE_CURVE ( 'NONE', #349, #13499, #15394, .T. ) ;
#11672=CARTESIAN_POINT ( 'NONE',  ( 5.000000000000000000, -26.12500000273118417, 0.000000000000000000 ) ) ;
#11676=DIRECTION ( 'NONE',  ( 1.000000000000000000, -0.000000000000000000, -1.239088197126290570E-16 ) ) ;
#11680=CARTESIAN_POINT ( 'NONE',  ( 1.846868145590736310, -23.62500000136559919, 4.458734124999999437 ) ) ;
#11684=CARTESIAN_POINT ( 'NONE',  ( 35.00000000000000000, 37.00000000000000000, -5.999999999999991118 ) ) ;
#11686=ORIENTED_EDGE ( 'NONE', *, *, #3443, .T. ) ;
#11687=CARTESIAN_POINT ( 'NONE',  ( -3.152801135295367985, -31.06250000136559564, 3.152801135295367096 ) ) ;
#11689=ORIENTED_EDGE ( 'NONE', *, *, #12701, .T. ) ;
#11694=CARTESIAN_POINT ( 'NONE',  ( 3.061616997868383141E-16, -27.75000000000000000, -5.000000000000000000 ) ) ;
#11698=CARTESIAN_POINT ( 'NONE',  ( -5.000000000000000888, -23.68750000273119127, -2.071067811865475949 ) ) ;
#11700=CARTESIAN_POINT ( 'NONE',  ( 3.152801135295366208, -25.56250000136559564, 3.152801135295367985 ) ) ;
#11707=LINE ( 'NONE', #7438, #11242 ) ;
#11708=EDGE_CURVE ( 'NONE', #3510, #12106, #10743, .T. ) ;
#11711=CARTESIAN_POINT ( 'NONE',  ( -4.458734124999999437, -27.18750000136559564, -5.460374474430324690E-16 ) ) ;
#11715=PRODUCT_CONTEXT ( 'NONE', #11438, 'mechanical' ) ;
#11720=EDGE_LOOP ( 'NONE', ( #1455, #8078 ) ) ;
#11724=PRODUCT_DEFINITION ( 'UNKNOWN', '', #6387, #13679 ) ;
#11746=CARTESIAN_POINT ( 'NONE',  ( 3.535533905932738197, -23.00000000273118772, -3.535533905932738197 ) ) ;
#11757=CARTESIAN_POINT ( 'NONE',  ( -3.152801135295367096, -28.31250000136559564, -3.152801135295367541 ) ) ;
#11767=CARTESIAN_POINT ( 'NONE',  ( 1.846868145590736310, -27.87500000136559564, 4.458734124999999437 ) ) ;
#11775=CARTESIAN_POINT ( 'NONE',  ( 3.535533905932736864, -24.12500000000000000, 3.535533905932738641 ) ) ;
#11780=CARTESIAN_POINT ( 'NONE',  ( -5.000000000000000000, -21.62500000273118772, -6.123233995736766282E-16 ) ) ;
#11782=CARTESIAN_POINT ( 'NONE',  ( 3.152801135295366208, -26.56250000136559564, 3.152801135295367985 ) ) ;
#11788=CARTESIAN_POINT ( 'NONE',  ( 2.071067811865492825, -28.93750000273118772, -4.999999999999983125 ) ) ;
#11794=CARTESIAN_POINT ( 'NONE',  ( 1.846868145590735200, -26.50000000136559208, -4.458734125000000326 ) ) ;
#11808=LINE ( 'NONE', #9327, #9425 ) ;
#11809=( BOUNDED_CURVE ( )  B_SPLINE_CURVE ( 2, ( #8068, #12963, #5706, #552, #13044, #1984, #15337, #4416, #4250 ),
 .UNSPECIFIED., .F., .F. ) 
 B_SPLINE_CURVE_WITH_KNOTS ( ( 3, 2, 2, 2, 3 ),
 ( 0.8750000000000000000, 0.8874999999999999556, 0.9000000000000001332, 0.9125000000000000888, 0.9250000000000002665 ),
 .UNSPECIFIED. ) 
 CURVE ( )  GEOMETRIC_REPRESENTATION_ITEM ( )  RATIONAL_B_SPLINE_CURVE ( ( 1.000000000000000000, 0.9238795325112867385, 1.000000000000000000, 0.9238795325112867385, 1.000000000000000000, 0.9238795325112867385, 1.000000000000000000, 0.9238795325112854062, 1.000000000000001332 ) ) 
 REPRESENTATION_ITEM ( '' )  );
#11824=ORIENTED_EDGE ( 'NONE', *, *, #601, .F. ) ;
#11825=CARTESIAN_POINT ( 'NONE',  ( 5.000000000000000000, -27.06250000000000000, 2.071067811865478614 ) ) ;
#11826=VERTEX_POINT ( 'NONE', #11301 ) ;
#11831=AXIS2_PLACEMENT_3D ( 'NONE', #10904, #15847, #4764 ) ;
#11834=CARTESIAN_POINT ( 'NONE',  ( 35.00000000000000000, 40.00000000000000000, -5.999999999999991118 ) ) ;
#11839=CARTESIAN_POINT ( 'NONE',  ( 6.000000000000000000, -13.00000000000000178, 1.500000000000000000 ) ) ;
#11841=CARTESIAN_POINT ( 'NONE',  ( 3.152801135295367541, -29.56250000136559208, -3.152801135295367541 ) ) ;
#11843=ORIENTED_EDGE ( 'NONE', *, *, #1593, .F. ) ;
#11849=CARTESIAN_POINT ( 'NONE',  ( 4.458734124999999437, -27.75000000136559564, 1.846868145590737864 ) ) ;
#11850=DIRECTION ( 'NONE',  ( -0.000000000000000000, 1.000000000000000000, -0.000000000000000000 ) ) ;
#11857=CARTESIAN_POINT ( 'NONE',  ( -9.184850993605147944E-16, -27.25000000000000000, 5.000000000000000000 ) ) ;
#11861=CARTESIAN_POINT ( 'NONE',  ( -8.190561711645485556E-16, -29.68750000136559208, 4.458734124999999437 ) ) ;
#11863=DIRECTION ( 'NONE',  ( -0.000000000000000000, 1.000000000000000000, -0.000000000000000000 ) ) ;
#11866=ORIENTED_EDGE ( 'NONE', *, *, #12068, .F. ) ;
#11869=CARTESIAN_POINT ( 'NONE',  ( -4.458734125000000326, -27.00000000136559208, -1.846868145590735644 ) ) ;
#11874=EDGE_CURVE ( 'NONE', #14954, #13586, #1914, .T. ) ;
#11875=CARTESIAN_POINT ( 'NONE',  ( -3.152801135295367096, -27.31250000136559564, -3.152801135295367541 ) ) ;
#11897=CARTESIAN_POINT ( 'NONE',  ( 0.000000000000000000, 0.000000000000000000, 0.000000000000000000 ) ) ;
#11899=DIRECTION ( 'NONE',  ( 0.000000000000000000, -1.000000000000000000, 0.000000000000000000 ) ) ;
#11902=CARTESIAN_POINT ( 'NONE',  ( 2.071067811865476394, -23.31250000273118772, 5.000000000000000000 ) ) ;
#11907=( BOUNDED_CURVE ( )  B_SPLINE_CURVE ( 2, ( #12187, #14316, #2342, #12117, #2031, #13092, #7285, #6977, #8347 ),
 .UNSPECIFIED., .F., .F. ) 
 B_SPLINE_CURVE_WITH_KNOTS ( ( 3, 2, 2, 2, 3 ),
 ( 0.07500000000000006661, 0.08750000000000007772, 0.1000000000000000888, 0.1125000000000000999, 0.1250000000000001110 ),
 .UNSPECIFIED. ) 
 CURVE ( )  GEOMETRIC_REPRESENTATION_ITEM ( )  RATIONAL_B_SPLINE_CURVE ( ( 0.9999999999999995559, 0.9238795325112871826, 1.000000000000000000, 0.9238795325112867385, 1.000000000000000000, 0.9238795325112867385, 1.000000000000000000, 0.9238795325112860723, 1.000000000000000666 ) ) 
 REPRESENTATION_ITEM ( '' )  );
#11915=CARTESIAN_POINT ( 'NONE',  ( -1.846868145590734756, -28.37500000136559564, -4.458734124999999437 ) ) ;
#11923=CARTESIAN_POINT ( 'NONE',  ( 3.152801135295366208, -27.81250000136559564, 3.152801135295367985 ) ) ;
#11925=EDGE_CURVE ( 'NONE', #10564, #4014, #15587, .T. ) ;
#11933=CARTESIAN_POINT ( 'NONE',  ( -4.458734125000000326, -30.00000000136559564, -1.846868145590735644 ) ) ;
#11935=CARTESIAN_POINT ( 'NONE',  ( 1.846868145590735200, -23.25000000136559564, -4.458734124999999437 ) ) ;
#11936=AXIS2_PLACEMENT_3D ( 'NONE', #3859, #8959, #13947 ) ;
#11938=ORIENTED_EDGE ( 'NONE', *, *, #7796, .T. ) ;
#11940=CARTESIAN_POINT ( 'NONE',  ( 6.000000000000000000, -13.00000000000000178, 1.500000000000000000 ) ) ;
#11941=CARTESIAN_POINT ( 'NONE',  ( -4.458734125000001214, -29.87500000136559564, 1.846868145590734089 ) ) ;
#11945=EDGE_CURVE ( 'NONE', #12106, #8217, #12902, .T. ) ;
#11950=CARTESIAN_POINT ( 'NONE',  ( 0.000000000000000000, 40.00000000000000000, 0.000000000000000000 ) ) ;
#11951=CARTESIAN_POINT ( 'NONE',  ( -4.458734124999999437, -28.18750000136559564, -5.460374474430324690E-16 ) ) ;
#11952=LINE ( 'NONE', #13241, #10382 ) ;
#11953=LINE ( 'NONE', #8279, #6428 ) ;
#11954=CARTESIAN_POINT ( 'NONE',  ( -3.535533905932738641, -30.50000000273118772, 3.535533905932737309 ) ) ;
#11972=DIRECTION ( 'NONE',  ( 0.000000000000000000, 0.000000000000000000, 1.000000000000000000 ) ) ;
#11978=CARTESIAN_POINT ( 'NONE',  ( -3.535533905932738641, -30.37500000000000000, 3.535533905932737309 ) ) ;
#11990=CARTESIAN_POINT ( 'NONE',  ( 1.846868145590735200, -30.50000000136559919, -4.458734124999999437 ) ) ;
#11992=VERTEX_POINT ( 'NONE', #5793 ) ;
#11995=VERTEX_POINT ( 'NONE', #3520 ) ;
#12000=CARTESIAN_POINT ( 'NONE',  ( 4.458734124999999437, -26.68750000136559564, 0.000000000000000000 ) ) ;
#12001=CYLINDRICAL_SURFACE ( 'NONE', #12015, 5.000000000000000000 ) ;
#12007=CARTESIAN_POINT ( 'NONE',  ( -2.071067811865475061, -23.68750000000000355, -5.000000000000000888 ) ) ;
#12014=CARTESIAN_POINT ( 'NONE',  ( -3.152801135295367096, -31.06250000136559564, -3.152801135295367541 ) ) ;
#12015=AXIS2_PLACEMENT_3D ( 'NONE', #3374, #8321, #951 ) ;
#12019=DIRECTION ( 'NONE',  ( -0.000000000000000000, 0.000000000000000000, 1.000000000000000000 ) ) ;
#12020=CARTESIAN_POINT ( 'NONE',  ( 4.458734124999999437, -29.43750000136559208, 0.000000000000000000 ) ) ;
#12021=DIRECTION ( 'NONE',  ( 0.000000000000000000, 0.000000000000000000, 1.000000000000000000 ) ) ;
#12024=CARTESIAN_POINT ( 'NONE',  ( -2.071067811865503483, -24.81250000273118772, -4.999999999999971578 ) ) ;
#12030=CARTESIAN_POINT ( 'NONE',  ( -1.846868145590734756, -24.37500000136559564, -4.458734125000000326 ) ) ;
#12045=CARTESIAN_POINT ( 'NONE',  ( -2.071067811865489272, -26.68750000000000000, -4.999999999999985789 ) ) ;
#12065=COLOUR_RGB ( '', 0.08235294, 0.09019608, 0.10196078) ;
#12068=EDGE_CURVE ( 'NONE', #11995, #2056, #14365, .T. ) ;
#12074=CARTESIAN_POINT ( 'NONE',  ( -3.152801135295367096, -29.31250000136559564, -3.152801135295367541 ) ) ;
#12076=ORIENTED_EDGE ( 'NONE', *, *, #5448, .F. ) ;
#12081=EDGE_LOOP ( 'NONE', ( #9898, #130, #539, #15490 ) ) ;
#12082=CARTESIAN_POINT ( 'NONE',  ( -3.152801135295367985, -27.06250000136559564, 3.152801135295367096 ) ) ;
#12086=EDGE_CURVE ( 'NONE', #10126, #8371, #426, .T. ) ;
#12094=CARTESIAN_POINT ( 'NONE',  ( -5.000000000000000888, -27.56250000000000000, -2.071067811865475949 ) ) ;
#12095=CARTESIAN_POINT ( 'NONE',  ( -2.071067811865475061, -21.81250000273118772, -5.000000000000000888 ) ) ;
#12096=( BOUNDED_CURVE ( )  B_SPLINE_CURVE ( 2, ( #2446, #4652, #8694, #2304, #1086, #9818, #4728, #49, #2216 ),
 .UNSPECIFIED., .F., .F. ) 
 B_SPLINE_CURVE_WITH_KNOTS ( ( 3, 2, 2, 2, 3 ),
 ( 0.7249999999999999778, 0.7375000000000000444, 0.7500000000000000000, 0.7624999999999999556, 0.7750000000000000222 ),
 .UNSPECIFIED. ) 
 CURVE ( )  GEOMETRIC_REPRESENTATION_ITEM ( )  RATIONAL_B_SPLINE_CURVE ( ( 1.000000000000000000, 0.9238795325112867385, 1.000000000000000000, 0.9238795325112867385, 1.000000000000000000, 0.9238795325112867385, 1.000000000000000000, 0.9238795325112867385, 1.000000000000000000 ) ) 
 REPRESENTATION_ITEM ( '' )  );
#12104=CARTESIAN_POINT ( 'NONE',  ( 4.458734125000000326, -27.37500000136559564, -1.846868145590734978 ) ) ;
#12106=VERTEX_POINT ( 'NONE', #7259 ) ;
#12110=ADVANCED_FACE ( 'NONE', ( #14686 ), #8554, .F. ) ;
#12114=CARTESIAN_POINT ( 'NONE',  ( 2.730187237215162345E-16, -22.43750000136559564, -4.458734124999999437 ) ) ;
#12115=FACE_OUTER_BOUND ( 'NONE', #4997, .T. ) ;
#12117=CARTESIAN_POINT ( 'NONE',  ( 5.000000000000000000, -31.06250000000000000, 2.071067811865478614 ) ) ;
#12125=EDGE_CURVE ( 'NONE', #9076, #2433, #8115, .T. ) ;
#12128=CARTESIAN_POINT ( 'NONE',  ( 5.000000000000000000, -28.06250000000000000, 2.071067811865478614 ) ) ;
#12140=ADVANCED_FACE ( 'NONE', ( #4904 ), #12001, .T. ) ;
#12144=CARTESIAN_POINT ( 'NONE',  ( -2.071067811865492381, -29.31250000000000000, 4.999999999999985789 ) ) ;
#12147=CARTESIAN_POINT ( 'NONE',  ( -2.071067811865456854, -29.43750000273118062, 5.000000000000021316 ) ) ;
#12151=CARTESIAN_POINT ( 'NONE',  ( 1.846868145590735200, -27.50000000136559564, -4.458734124999999437 ) ) ;
#12153=DIRECTION ( 'NONE',  ( 0.000000000000000000, 0.000000000000000000, 1.000000000000000000 ) ) ;
#12158=CARTESIAN_POINT ( 'NONE',  ( -3.152801135295367985, -24.06250000136559564, 3.152801135295367096 ) ) ;
#12159=CARTESIAN_POINT ( 'NONE',  ( -5.000000000000000888, -23.68750000273119127, -2.071067811865475949 ) ) ;
#12162=CARTESIAN_POINT ( 'NONE',  ( 0.000000000000000000, -20.00000000000000000, 0.000000000000000000 ) ) ;
#12168=CARTESIAN_POINT ( 'NONE',  ( 3.152801135295366208, -26.56250000136559564, 3.152801135295367985 ) ) ;
#12175=CARTESIAN_POINT ( 'NONE',  ( 4.458734124999999437, -25.50000000136559919, 1.846868145590737864 ) ) ;
#12181=CARTESIAN_POINT ( 'NONE',  ( 5.000000000000000000, -22.06250000000000000, 2.071067811865478614 ) ) ;
#12184=CARTESIAN_POINT ( 'NONE',  ( -1.846868145590737420, -25.00000000136559564, 4.458734124999999437 ) ) ;
#12187=CARTESIAN_POINT ( 'NONE',  ( -9.184850993605147944E-16, -31.25000000000000000, 5.000000000000000888 ) ) ;
#12188=LINE ( 'NONE', #9938, #14012 ) ;
#12194=ORIENTED_EDGE ( 'NONE', *, *, #1593, .T. ) ;
#12222=EDGE_CURVE ( 'NONE', #6666, #79, #3764, .T. ) ;
#12224=CARTESIAN_POINT ( 'NONE',  ( -1.846868145590734756, -24.37500000136559564, -4.458734124999999437 ) ) ;
#12226=VECTOR ( 'NONE', #2546, 1000.000000000000000 ) ;
#12227=CARTESIAN_POINT ( 'NONE',  ( -4.458734124999999437, -22.93750000136559564, -5.460374474430324690E-16 ) ) ;
#12231=ORIENTED_EDGE ( 'NONE', *, *, #12522, .F. ) ;
#12235=CARTESIAN_POINT ( 'NONE',  ( -1.846868145590737420, -24.00000000136559564, 4.458734124999999437 ) ) ;
#12242=CARTESIAN_POINT ( 'NONE',  ( -3.535533905932738641, -22.37500000000000000, 3.535533905932737309 ) ) ;
#12246=CARTESIAN_POINT ( 'NONE',  ( -1.846868145590734756, -28.12500000136559564, -4.458734125000000326 ) ) ;
#12252=DIRECTION ( 'NONE',  ( 0.000000000000000000, 0.000000000000000000, 1.000000000000000000 ) ) ;
#12254=ORIENTED_EDGE ( 'NONE', *, *, #11708, .T. ) ;
#12257=CARTESIAN_POINT ( 'NONE',  ( -1.846868145590734756, -25.12500000136559564, -4.458734125000000326 ) ) ;
#12266=CARTESIAN_POINT ( 'NONE',  ( 2.730187237215162345E-16, -24.43750000136559564, -4.458734124999999437 ) ) ;
#12267=AXIS2_PLACEMENT_3D ( 'NONE', #4356, #2000, #3299 ) ;
#12270=CARTESIAN_POINT ( 'NONE',  ( 2.071067811865475505, -29.93750000273118417, -5.000000000000000888 ) ) ;
#12273=CARTESIAN_POINT ( 'NONE',  ( 2.730187237215162345E-16, -31.18750000136559564, -4.458734124999999437 ) ) ;
#12276=( GEOMETRIC_REPRESENTATION_CONTEXT ( 3 ) GLOBAL_UNCERTAINTY_ASSIGNED_CONTEXT ( ( #6103 ) ) GLOBAL_UNIT_ASSIGNED_CONTEXT ( ( #10053, #6659, #7954 ) ) REPRESENTATION_CONTEXT ( 'NONE', 'WORKASPACE' ) );
#12280=ORIENTED_EDGE ( 'NONE', *, *, #13644, .T. ) ;
#12296=EDGE_LOOP ( 'NONE', ( #483, #6134, #11665, #4445 ) ) ;
#12300=ADVANCED_FACE ( 'NONE', ( #6363 ), #12477, .T. ) ;
#12302=CARTESIAN_POINT ( 'NONE',  ( -3.535533905932737309, -29.62500000000000355, -3.535533905932738197 ) ) ;
#12303=FACE_OUTER_BOUND ( 'NONE', #594, .T. ) ;
#12305=FACE_OUTER_BOUND ( 'NONE', #13538, .T. ) ;
#12308=CARTESIAN_POINT ( 'NONE',  ( -9.184850993605147944E-16, -28.37500000273118772, 5.000000000000000000 ) ) ;
#12309=CARTESIAN_POINT ( 'NONE',  ( -4.458734125000000326, -27.12500000136559564, 1.846868145590734089 ) ) ;
#12310=CARTESIAN_POINT ( 'NONE',  ( -1.846868145590734756, -23.12500000136559564, -4.458734124999999437 ) ) ;
#12312=AXIS2_PLACEMENT_3D ( 'NONE', #10915, #14403, #5828 ) ;
#12313=VECTOR ( 'NONE', #2284, 1000.000000000000000 ) ;
#12319=CARTESIAN_POINT ( 'NONE',  ( 2.730187237215162345E-16, -22.43750000136559564, -4.458734124999999437 ) ) ;
#12321=DIRECTION ( 'NONE',  ( 0.000000000000000000, 0.000000000000000000, -1.000000000000000000 ) ) ;
#12331=LINE ( 'NONE', #10969, #611 ) ;
#12333=CARTESIAN_POINT ( 'NONE',  ( -4.458734124999999437, -27.93750000136559564, -5.460374474430324690E-16 ) ) ;
#12337=ORIENTED_EDGE ( 'NONE', *, *, #7117, .F. ) ;
#12338=ORIENTED_EDGE ( 'NONE', *, *, #11925, .T. ) ;
#12341=CIRCLE ( 'NONE', #5390, 2.649999999999992806 ) ;
#12342=CARTESIAN_POINT ( 'NONE',  ( 1.846868145590735200, -23.25000000136559208, -4.458734125000000326 ) ) ;
#12347=AXIS2_PLACEMENT_3D ( 'NONE', #7826, #6605, #1663 ) ;
#12354=CARTESIAN_POINT ( 'NONE',  ( 4.458734124999999437, -24.75000000136559564, 1.846868145590737864 ) ) ;
#12357=CARTESIAN_POINT ( 'NONE',  ( 2.071067811865476394, -28.31250000273118772, 5.000000000000000000 ) ) ;
#12359=CARTESIAN_POINT ( 'NONE',  ( 2.730187237215162345E-16, -29.18750000136559208, -4.458734124999999437 ) ) ;
#12361=ORIENTED_EDGE ( 'NONE', *, *, #2364, .T. ) ;
#12376=ADVANCED_FACE ( 'NONE', ( #10637 ), #1978, .T. ) ;
#12390=CARTESIAN_POINT ( 'NONE',  ( -3.152801135295367985, -24.06250000136559564, 3.152801135295367096 ) ) ;
#12392=CARTESIAN_POINT ( 'NONE',  ( 2.730187237215162345E-16, -22.18750000136559564, -4.458734124999999437 ) ) ;
#12400=CARTESIAN_POINT ( 'NONE',  ( -1.846868145590737420, -23.00000000136559564, 4.458734124999999437 ) ) ;
#12410=CARTESIAN_POINT ( 'NONE',  ( 3.152801135295366208, -27.56250000136559564, 3.152801135295367985 ) ) ;
#12412=VERTEX_POINT ( 'NONE', #6924 ) ;
#12414=VERTEX_POINT ( 'NONE', #12718 ) ;
#12416=ADVANCED_FACE ( 'NONE', ( #11668 ), #6839, .T. ) ;
#12419=CARTESIAN_POINT ( 'NONE',  ( -4.458734125000001214, -25.87500000136559919, 1.846868145590734089 ) ) ;
#12428=CARTESIAN_POINT ( 'NONE',  ( -3.535533905932738641, -28.37500000000000000, 3.535533905932737309 ) ) ;
#12430=CARTESIAN_POINT ( 'NONE',  ( 3.535533905932736864, -30.25000000273118417, 3.535533905932738641 ) ) ;
#12431=DIRECTION ( 'NONE',  ( -0.000000000000000000, 1.000000000000000000, -0.000000000000000000 ) ) ;
#12432=CARTESIAN_POINT ( 'NONE',  ( -1.846868145590734756, -29.12500000136559564, -4.458734124999999437 ) ) ;
#12435=EDGE_LOOP ( 'NONE', ( #15763, #9034, #7094, #8750, #14427 ) ) ;
#12443=CARTESIAN_POINT ( 'NONE',  ( 3.152801135295367541, -31.56250000136559564, -3.152801135295367541 ) ) ;
#12448=FACE_OUTER_BOUND ( 'NONE', #10700, .T. ) ;
#12451=DIRECTION ( 'NONE',  ( -0.000000000000000000, 1.000000000000000000, -0.000000000000000000 ) ) ;
#12452=EDGE_CURVE ( 'NONE', #2123, #6666, #14888, .T. ) ;
#12456=DIRECTION ( 'NONE',  ( -0.000000000000000000, -1.000000000000000000, -0.000000000000000000 ) ) ;
#12462=DIRECTION ( 'NONE',  ( 0.000000000000000000, 0.000000000000000000, 1.000000000000000000 ) ) ;
#12465=CARTESIAN_POINT ( 'NONE',  ( 5.000000000000000888, -28.06250000273118772, -2.071067811865475505 ) ) ;
#12466=CARTESIAN_POINT ( 'NONE',  ( -3.152801135295367985, -25.06250000136559564, 3.152801135295367096 ) ) ;
#12475=ORIENTED_EDGE ( 'NONE', *, *, #13884, .T. ) ;
#12477=CYLINDRICAL_SURFACE ( 'NONE', #14375, 5.000000000000000000 ) ;
#12480=CARTESIAN_POINT ( 'NONE',  ( 5.000000000000000888, -25.93750000000000711, -2.071067811865475505 ) ) ;
#12487=CARTESIAN_POINT ( 'NONE',  ( 1.846868145590735200, -27.25000000136559564, -4.458734125000000326 ) ) ;
#12494=CARTESIAN_POINT ( 'NONE',  ( 1.846868145590735200, -24.25000000136559564, -4.458734125000000326 ) ) ;
#12499=EDGE_CURVE ( 'NONE', #11995, #4136, #9948, .T. ) ;
#12501=CYLINDRICAL_SURFACE ( 'NONE', #12967, 5.000000000000000000 ) ;
#12503=CARTESIAN_POINT ( 'NONE',  ( -3.535533905932737309, -28.62500000000000000, -3.535533905932738197 ) ) ;
#12507=CARTESIAN_POINT ( 'NONE',  ( 3.535533905932738197, -29.00000000273118772, -3.535533905932738197 ) ) ;
#12510=CARTESIAN_POINT ( 'NONE',  ( -4.458734125000000326, -28.87500000136559564, 1.846868145590734089 ) ) ;
#12517=CYLINDRICAL_SURFACE ( 'NONE', #15674, 5.000000000000000000 ) ;
#12521=DIRECTION ( 'NONE',  ( -0.000000000000000000, -1.000000000000000000, -0.000000000000000000 ) ) ;
#12522=EDGE_CURVE ( 'NONE', #4598, #2810, #12541, .T. ) ;
#12523=CARTESIAN_POINT ( 'NONE',  ( 2.730187237215162345E-16, -31.43750000136559564, -4.458734124999999437 ) ) ;
#12525=AXIS2_PLACEMENT_3D ( 'NONE', #11684, #12731, #5403 ) ;
#12527=DIRECTION ( 'NONE',  ( 0.000000000000000000, 1.000000000000000000, 0.000000000000000000 ) ) ;
#12534=FACE_OUTER_BOUND ( 'NONE', #3660, .T. ) ;
#12541=CIRCLE ( 'NONE', #15926, 6.000000000000000888 ) ;
#12551=CARTESIAN_POINT ( 'NONE',  ( -3.152801135295367985, -23.06250000136559564, 3.152801135295367096 ) ) ;
#12564=EDGE_CURVE ( 'NONE', #13455, #8371, #5105, .T. ) ;
#12572=CARTESIAN_POINT ( 'NONE',  ( -4.458734125000001214, -23.87500000136559564, 1.846868145590734089 ) ) ;
#12574=EDGE_LOOP ( 'NONE', ( #13727, #7918, #8198, #13837 ) ) ;
#12579=CARTESIAN_POINT ( 'NONE',  ( 3.152801135295366208, -29.81250000136559208, 3.152801135295367985 ) ) ;
#12590=CARTESIAN_POINT ( 'NONE',  ( 5.000000000000000888, -29.93750000000000355, -2.071067811865475505 ) ) ;
#12592=DIRECTION ( 'NONE',  ( -0.000000000000000000, -1.000000000000000000, -0.000000000000000000 ) ) ;
#12593=CARTESIAN_POINT ( 'NONE',  ( -5.000000000000000888, -29.68750000273118772, -2.071067811865475949 ) ) ;
#12595=CARTESIAN_POINT ( 'NONE',  ( 4.458734124999999437, -31.37500000136559564, -1.846868145590734978 ) ) ;
#12608=CARTESIAN_POINT ( 'NONE',  ( -3.152801135295367096, -30.31250000136559564, -3.152801135295367541 ) ) ;
#12614=( BOUNDED_CURVE ( )  B_SPLINE_CURVE ( 2, ( #10622, #7807, #15866, #12128, #2353, #3483, #1141, #7300, #836 ),
 .UNSPECIFIED., .F., .F. ) 
 B_SPLINE_CURVE_WITH_KNOTS ( ( 3, 2, 2, 2, 3 ),
 ( 0.3750000000000000000, 0.3875000000000000111, 0.4000000000000000222, 0.4125000000000000333, 0.4250000000000000444 ),
 .UNSPECIFIED. ) 
 CURVE ( )  GEOMETRIC_REPRESENTATION_ITEM ( )  RATIONAL_B_SPLINE_CURVE ( ( 1.000000000000000000, 0.9238795325112867385, 1.000000000000000000, 0.9238795325112867385, 1.000000000000000000, 0.9238795325112867385, 1.000000000000000000, 0.9238795325112864054, 1.000000000000000444 ) ) 
 REPRESENTATION_ITEM ( '' )  );
#12615=CARTESIAN_POINT ( 'NONE',  ( 0.000000000000000000, -20.00000000000000000, 5.000000000000000000 ) ) ;
#12626=CYLINDRICAL_SURFACE ( 'NONE', #9731, 5.000000000000000000 ) ;
#12630=CARTESIAN_POINT ( 'NONE',  ( 2.071067811865482611, -27.93750000273118772, -4.999999999999992895 ) ) ;
#12631=CARTESIAN_POINT ( 'NONE',  ( 4.458734124999997661, -22.75000000136559919, 1.846868145590737864 ) ) ;
#12633=CARTESIAN_POINT ( 'NONE',  ( 0.000000000000000000, 20.00000000000000000, 0.000000000000000000 ) ) ;
#12646=CARTESIAN_POINT ( 'NONE',  ( 5.000000000000000000, -26.06250000000000355, 2.071067811865478614 ) ) ;
#12648=LINE ( 'NONE', #2551, #5904 ) ;
#12652=CARTESIAN_POINT ( 'NONE',  ( 4.458734124999999437, -21.50000000136559208, 1.846868145590737864 ) ) ;
#12657=VERTEX_POINT ( 'NONE', #5188 ) ;
#12659=CARTESIAN_POINT ( 'NONE',  ( 4.458734124999999437, -22.43750000136559564, 0.000000000000000000 ) ) ;
#12662=CARTESIAN_POINT ( 'NONE',  ( -5.000000000000000888, -28.43750000000000355, 2.071067811865474617 ) ) ;
#12664=CARTESIAN_POINT ( 'NONE',  ( 0.000000000000000000, -13.00000000000000178, 1.500000000000000000 ) ) ;
#12665=DIRECTION ( 'NONE',  ( 0.000000000000000000, 0.000000000000000000, 1.000000000000000000 ) ) ;
#12666=CARTESIAN_POINT ( 'NONE',  ( -2.071067811865478170, -29.31250000000000000, 5.000000000000000000 ) ) ;
#12668=CARTESIAN_POINT ( 'NONE',  ( 6.000000000000000000, -13.00000000000000178, 0.000000000000000000 ) ) ;
#12669=CARTESIAN_POINT ( 'NONE',  ( 5.000000000000000888, -26.06250000273118417, -2.071067811865475505 ) ) ;
#12670=CARTESIAN_POINT ( 'NONE',  ( 4.458734124999999437, -26.43750000136559564, 0.000000000000000000 ) ) ;
#12672=ORIENTED_EDGE ( 'NONE', *, *, #11368, .T. ) ;
#12690=VERTEX_POINT ( 'NONE', #7946 ) ;
#12692=CARTESIAN_POINT ( 'NONE',  ( 0.000000000000000000, -11.00000000000000178, 0.000000000000000000 ) ) ;
#12701=EDGE_CURVE ( 'NONE', #4620, #12414, #1462, .T. ) ;
#12704=CARTESIAN_POINT ( 'NONE',  ( -2.071067811865489272, -23.68749999999999645, -4.999999999999985789 ) ) ;
#12707=ORIENTED_EDGE ( 'NONE', *, *, #14247, .T. ) ;
#12713=VECTOR ( 'NONE', #6628, 1000.000000000000000 ) ;
#12718=CARTESIAN_POINT ( 'NONE',  ( -9.184850993605147944E-16, -25.25000000000000000, 5.000000000000000000 ) ) ;
#12724=FACE_OUTER_BOUND ( 'NONE', #5296, .T. ) ;
#12728=CARTESIAN_POINT ( 'NONE',  ( 1.846868145590735200, -23.25000000136559208, -4.458734125000000326 ) ) ;
#12731=DIRECTION ( 'NONE',  ( -1.239088197126290570E-16, 0.000000000000000000, -1.000000000000000000 ) ) ;
#12734=CARTESIAN_POINT ( 'NONE',  ( -4.458734124999999437, -30.18750000136559564, -5.460374474430324690E-16 ) ) ;
#12741=FACE_OUTER_BOUND ( 'NONE', #9848, .T. ) ;
#12742=CARTESIAN_POINT ( 'NONE',  ( 0.000000000000000000, -20.00000000000000000, 5.000000000000000000 ) ) ;
#12743=ADVANCED_FACE ( 'NONE', ( #4127 ), #6649, .F. ) ;
#12744=CARTESIAN_POINT ( 'NONE',  ( -5.000000000000000000, -29.50000000000000355, -6.123233995736766282E-16 ) ) ;
#12748=CARTESIAN_POINT ( 'NONE',  ( 3.535533905932738197, -26.00000000273118417, -3.535533905932738197 ) ) ;
#12750=CARTESIAN_POINT ( 'NONE',  ( -1.846868145590734756, -25.12500000136559564, -4.458734124999999437 ) ) ;
#12761=ADVANCED_FACE ( 'NONE', ( #15295 ), #12517, .T. ) ;
#12762=CARTESIAN_POINT ( 'NONE',  ( 4.458734124999999437, -29.68750000136559208, 0.000000000000000000 ) ) ;
#12771=CARTESIAN_POINT ( 'NONE',  ( 2.730187237215162345E-16, -30.18750000136559564, -4.458734124999999437 ) ) ;
#12776=CARTESIAN_POINT ( 'NONE',  ( 35.00000000000000000, 37.00000000000000000, -5.999999999999991118 ) ) ;
#12777=CIRCLE ( 'NONE', #6885, 2.649999999999985700 ) ;
#12783=CARTESIAN_POINT ( 'NONE',  ( 1.846868145590735200, -22.50000000136559564, -4.458734124999999437 ) ) ;
#12793=ORIENTED_EDGE ( 'NONE', *, *, #446, .F. ) ;
#12797=EDGE_CURVE ( 'NONE', #12657, #2074, #6884, .T. ) ;
#12798=AXIS2_PLACEMENT_3D ( 'NONE', #548, #10476, #15494 ) ;
#12802=AXIS2_PLACEMENT_3D ( 'NONE', #5468, #7987, #5392 ) ;
#12808=CARTESIAN_POINT ( 'NONE',  ( 4.458734125000000326, -23.37500000136559564, -1.846868145590734978 ) ) ;
#12813=ORIENTED_EDGE ( 'NONE', *, *, #9578, .T. ) ;
#12816=CARTESIAN_POINT ( 'NONE',  ( -1.846868145590737420, -31.00000000136559564, 4.458734124999999437 ) ) ;
#12826=CARTESIAN_POINT ( 'NONE',  ( -9.184850993605147944E-16, -25.25000000000000000, 5.000000000000000000 ) ) ;
#12830=DIRECTION ( 'NONE',  ( 0.000000000000000000, 1.000000000000000000, 0.000000000000000000 ) ) ;
#12831=CARTESIAN_POINT ( 'NONE',  ( -2.071067811865475061, -25.81250000273118417, -5.000000000000000888 ) ) ;
#12833=CARTESIAN_POINT ( 'NONE',  ( -3.152801135295367985, -24.81250000136559564, 3.152801135295367096 ) ) ;
#12836=VERTEX_POINT ( 'NONE', #3158 ) ;
#12837=CARTESIAN_POINT ( 'NONE',  ( 3.061616997868383141E-16, -28.87500000273118772, -5.000000000000000000 ) ) ;
#12840=CARTESIAN_POINT ( 'NONE',  ( 5.000000000000000888, -29.06250000273118772, -2.071067811865475505 ) ) ;
#12843=ORIENTED_EDGE ( 'NONE', *, *, #11418, .F. ) ;
#12848=CARTESIAN_POINT ( 'NONE',  ( 3.152801135295366208, -28.81250000136559564, 3.152801135295367985 ) ) ;
#12860=CARTESIAN_POINT ( 'NONE',  ( -4.458734125000001214, -28.87500000136559564, 1.846868145590734089 ) ) ;
#12867=DIRECTION ( 'NONE',  ( 0.000000000000000000, -0.000000000000000000, 1.000000000000000000 ) ) ;
#12873=CARTESIAN_POINT ( 'NONE',  ( 1.846868145590735200, -23.50000000136559564, -4.458734124999999437 ) ) ;
#12883=CARTESIAN_POINT ( 'NONE',  ( -2.071067811865456854, -30.31249999999999645, 5.000000000000021316 ) ) ;
#12891=LINE ( 'NONE', #11839, #2149 ) ;
#12893=CARTESIAN_POINT ( 'NONE',  ( 3.535533905932738197, -25.00000000273118417, -3.535533905932738197 ) ) ;
#12895=CARTESIAN_POINT ( 'NONE',  ( -3.152801135295367096, -23.06250000136559564, -3.152801135295367541 ) ) ;
#12898=LINE ( 'NONE', #5557, #13548 ) ;
#12900=EDGE_LOOP ( 'NONE', ( #12672, #2940, #2891, #14949 ) ) ;
#12901=CARTESIAN_POINT ( 'NONE',  ( -1.846868145590734756, -29.37500000136559564, -4.458734125000000326 ) ) ;
#12902=LINE ( 'NONE', #720, #15135 ) ;
#12903=ORIENTED_EDGE ( 'NONE', *, *, #7781, .T. ) ;
#12908=CARTESIAN_POINT ( 'NONE',  ( 3.061616997868383141E-16, -26.75000000000000000, -5.000000000000000000 ) ) ;
#12913=CARTESIAN_POINT ( 'NONE',  ( 5.000000000000000000, -24.12500000273118772, 0.000000000000000000 ) ) ;
#12915=CARTESIAN_POINT ( 'NONE',  ( -8.190561711645485556E-16, -26.68750000136559564, 4.458734124999999437 ) ) ;
#12925=CARTESIAN_POINT ( 'NONE',  ( -8.190561711645485556E-16, -25.93750000136559564, 4.458734124999999437 ) ) ;
#12932=CARTESIAN_POINT ( 'NONE',  ( 3.535533905932738197, -31.87500000000000000, -3.535533905932738197 ) ) ;
#12937=ORIENTED_EDGE ( 'NONE', *, *, #3213, .F. ) ;
#12957=CARTESIAN_POINT ( 'NONE',  ( 5.000000000000000000, -23.12500000273118772, 0.000000000000000000 ) ) ;
#12963=CARTESIAN_POINT ( 'NONE',  ( 2.071067811865476394, -23.18749999999999645, 5.000000000000000000 ) ) ;
#12967=AXIS2_PLACEMENT_3D ( 'NONE', #5248, #7603, #12665 ) ;
#12969=CARTESIAN_POINT ( 'NONE',  ( -4.458734125000000326, -29.12500000136559564, 1.846868145590734089 ) ) ;
#12977=CARTESIAN_POINT ( 'NONE',  ( 4.458734124999999437, -25.68750000136559564, 0.000000000000000000 ) ) ;
#12984=CARTESIAN_POINT ( 'NONE',  ( 5.000000000000000000, -26.00000000000000355, 0.000000000000000000 ) ) ;
#12988=CARTESIAN_POINT ( 'NONE',  ( 4.458734125000000326, -29.37500000136559208, -1.846868145590734978 ) ) ;
#12990=CARTESIAN_POINT ( 'NONE',  ( 1.846868145590735200, -28.25000000136559919, -4.458734124999999437 ) ) ;
#12991=APPLICATION_CONTEXT ( 'automotive_design' ) ;
#13000=EDGE_CURVE ( 'NONE', #3510, #4663, #7354, .T. ) ;
#13003=CARTESIAN_POINT ( 'NONE',  ( -4.458734125000000326, -29.25000000136559564, -1.846868145590735644 ) ) ;
#13004=DIRECTION ( 'NONE',  ( 0.000000000000000000, 0.000000000000000000, 1.000000000000000000 ) ) ;
#13013=VECTOR ( 'NONE', #14999, 1000.000000000000000 ) ;
#13017=VECTOR ( 'NONE', #5153, 1000.000000000000000 ) ;
#13022=VECTOR ( 'NONE', #4232, 1000.000000000000000 ) ;
#13026=CARTESIAN_POINT ( 'NONE',  ( 2.071067811865475505, -24.81250000000000000, -5.000000000000000888 ) ) ;
#13037=( BOUNDED_CURVE ( )  B_SPLINE_CURVE ( 2, ( #6468, #7771, #11380, #331, #10180, #12662, #1602, #14218, #9211 ),
 .UNSPECIFIED., .F., .F. ) 
 B_SPLINE_CURVE_WITH_KNOTS ( ( 3, 2, 2, 2, 3 ),
 ( 0.3249999999999999556, 0.3374999999999999667, 0.3499999999999999778, 0.3624999999999999889, 0.3750000000000000000 ),
 .UNSPECIFIED. ) 
 CURVE ( )  GEOMETRIC_REPRESENTATION_ITEM ( )  RATIONAL_B_SPLINE_CURVE ( ( 1.000000000000000444, 0.9238795325112864054, 1.000000000000000000, 0.9238795325112867385, 1.000000000000000000, 0.9238795325112867385, 1.000000000000000000, 0.9238795325112867385, 1.000000000000000000 ) ) 
 REPRESENTATION_ITEM ( '' )  );
#13044=CARTESIAN_POINT ( 'NONE',  ( 5.000000000000000000, -23.00000000000000000, 0.000000000000000000 ) ) ;
#13046=DIRECTION ( 'NONE',  ( -1.000000000000000000, 0.000000000000000000, 1.239088197126290570E-16 ) ) ;
#13048=CARTESIAN_POINT ( 'NONE',  ( -1.846868145590737420, -28.00000000136559564, 4.458734124999997661 ) ) ;
#13059=CARTESIAN_POINT ( 'NONE',  ( 4.458734125000000326, -26.62500000136559564, -1.846868145590734978 ) ) ;
#13067=AXIS2_PLACEMENT_3D ( 'NONE', #7898, #14019, #5387 ) ;
#13068=CARTESIAN_POINT ( 'NONE',  ( -5.000000000000000888, -25.56250000000000355, -2.071067811865475949 ) ) ;
#13072=DIRECTION ( 'NONE',  ( -0.000000000000000000, -1.000000000000000000, -0.000000000000000000 ) ) ;
#13073=CARTESIAN_POINT ( 'NONE',  ( 4.458734124999999437, -30.50000000136559919, 1.846868145590737864 ) ) ;
#13075=FACE_OUTER_BOUND ( 'NONE', #8356, .T. ) ;
#13082=CARTESIAN_POINT ( 'NONE',  ( 2.071067811865497710, -29.31250000273118062, 4.999999999999978684 ) ) ;
#13088=CARTESIAN_POINT ( 'NONE',  ( 4.458734124999999437, -26.68750000136559564, 0.000000000000000000 ) ) ;
#13092=CARTESIAN_POINT ( 'NONE',  ( 5.000000000000000888, -30.93750000000000355, -2.071067811865475505 ) ) ;
#13102=VECTOR ( 'NONE', #5030, 1000.000000000000000 ) ;
#13109=LINE ( 'NONE', #14638, #7359 ) ;
#13118=VERTEX_POINT ( 'NONE', #13395 ) ;
#13130=ADVANCED_FACE ( 'NONE', ( #2333, #4849, #9772 ), #6145, .T. ) ;
#13133=CARTESIAN_POINT ( 'NONE',  ( 1.846868145590735200, -29.50000000136559564, -4.458734124999999437 ) ) ;
#13143=CARTESIAN_POINT ( 'NONE',  ( 1.846868145590736310, -26.87500000136559208, 4.458734124999999437 ) ) ;
#13146=CARTESIAN_POINT ( 'NONE',  ( -2.071067811865499486, -29.68750000000000000, -4.999999999999975131 ) ) ;
#13149=CARTESIAN_POINT ( 'NONE',  ( -5.000000000000000888, -26.43750000000000355, 2.071067811865474617 ) ) ;
#13153=CARTESIAN_POINT ( 'NONE',  ( -1.846868145590734756, -31.12500000136559564, -4.458734125000000326 ) ) ;
#13156=CARTESIAN_POINT ( 'NONE',  ( 1.846868145590735200, -24.25000000136559564, -4.458734124999999437 ) ) ;
#13161=CARTESIAN_POINT ( 'NONE',  ( 2.730187237215162345E-16, -29.18750000136559208, -4.458734124999999437 ) ) ;
#13162=CARTESIAN_POINT ( 'NONE',  ( 5.000000000000000000, -29.12500000273118772, 0.000000000000000000 ) ) ;
#13163=ORIENTED_EDGE ( 'NONE', *, *, #13234, .F. ) ;
#13167=CARTESIAN_POINT ( 'NONE',  ( 1.846868145590736310, -26.87500000136559208, 4.458734124999999437 ) ) ;
#13170=CARTESIAN_POINT ( 'NONE',  ( 5.000000000000000888, -31.06250000273118417, -2.071067811865475505 ) ) ;
#13183=CARTESIAN_POINT ( 'NONE',  ( 5.000000000000000000, -22.12500000273118417, 0.000000000000000000 ) ) ;
#13184=ORIENTED_EDGE ( 'NONE', *, *, #5019, .T. ) ;
#13194=LINE ( 'NONE', #3663, #13264 ) ;
#13199=CARTESIAN_POINT ( 'NONE',  ( -3.535533905932737309, -29.75000000273118417, -3.535533905932738197 ) ) ;
#13202=CARTESIAN_POINT ( 'NONE',  ( -1.846868145590737420, -30.00000000136559919, 4.458734124999997661 ) ) ;
#13209=CARTESIAN_POINT ( 'NONE',  ( 3.152801135295366208, -28.81250000136559564, 3.152801135295367985 ) ) ;
#13210=CARTESIAN_POINT ( 'NONE',  ( -35.00000000000000000, 37.00000000000000000, 0.000000000000000000 ) ) ;
#13213=EDGE_CURVE ( 'NONE', #14496, #13118, #13037, .T. ) ;
#13214=CIRCLE ( 'NONE', #6274, 25.00000000000000000 ) ;
#13215=AXIS2_PLACEMENT_3D ( 'NONE', #15651, #5469, #9195 ) ;
#13218=CARTESIAN_POINT ( 'NONE',  ( 3.061616997868383141E-16, -22.75000000000000000, -5.000000000000000000 ) ) ;
#13223=CARTESIAN_POINT ( 'NONE',  ( 2.071067811865476394, -21.31250000273118772, 5.000000000000000000 ) ) ;
#13229=CARTESIAN_POINT ( 'NONE',  ( 3.061616997868383141E-16, -27.87500000273118772, -5.000000000000000000 ) ) ;
#13230=CARTESIAN_POINT ( 'NONE',  ( 2.730187237215162345E-16, -28.18750000136559564, -4.458734124999999437 ) ) ;
#13232=ORIENTED_EDGE ( 'NONE', *, *, #907, .T. ) ;
#13234=EDGE_CURVE ( 'NONE', #14535, #10378, #14369, .T. ) ;
#13240=CARTESIAN_POINT ( 'NONE',  ( 4.458734124999999437, -23.68750000136559564, 0.000000000000000000 ) ) ;
#13241=CARTESIAN_POINT ( 'NONE',  ( 35.00000000000000000, 40.00000000000000000, -5.999999999999991118 ) ) ;
#13249=ADVANCED_FACE ( 'NONE', ( #8322 ), #10589, .T. ) ;
#13258=CARTESIAN_POINT ( 'NONE',  ( -5.000000000000000888, -22.43749999999999645, 2.071067811865474617 ) ) ;
#13264=VECTOR ( 'NONE', #15964, 1000.000000000000000 ) ;
#13272=VECTOR ( 'NONE', #603, 1000.000000000000000 ) ;
#13273=CARTESIAN_POINT ( 'NONE',  ( 3.061616997868383141E-16, -29.87500000273118417, -5.000000000000000000 ) ) ;
#13276=CARTESIAN_POINT ( 'NONE',  ( 3.152801135295367541, -31.56250000136559564, -3.152801135295367541 ) ) ;
#13278=ORIENTED_EDGE ( 'NONE', *, *, #15093, .T. ) ;
#13279=DIRECTION ( 'NONE',  ( -0.000000000000000000, -1.000000000000000000, -0.000000000000000000 ) ) ;
#13285=EDGE_LOOP ( 'NONE', ( #3247, #9286, #10112, #3865 ) ) ;
#13286=CARTESIAN_POINT ( 'NONE',  ( -1.846868145590737420, -26.00000000136559564, 4.458734124999999437 ) ) ;
#13289=CARTESIAN_POINT ( 'NONE',  ( 3.535533905932738197, -30.00000000273118417, -3.535533905932738197 ) ) ;
#13292=CARTESIAN_POINT ( 'NONE',  ( -2.071067811865478170, -22.31250000000000000, 5.000000000000000000 ) ) ;
#13297=CARTESIAN_POINT ( 'NONE',  ( 5.000000000000000000, -21.12500000273118772, 0.000000000000000000 ) ) ;
#13298=AXIS2_PLACEMENT_3D ( 'NONE', #165, #1354, #5081 ) ;
#13306=CARTESIAN_POINT ( 'NONE',  ( 1.846868145590736310, -30.62500000136559208, 4.458734124999999437 ) ) ;
#13312=CLOSED_SHELL ( 'NONE', ( #12110, #14529, #11416, #13555, #10250, #6423, #9534, #7851, #12376, #870, #13249, #5844, #14445, #12300, #12140, #422, #1365, #2951, #9685, #12416, #5040, #7975, #7607, #164, #12761, #4743, #2240, #5902, #13130, #9923, #7648, #5961, #13712, #10217, #4406, #13595, #5603, #4626, #13907, #6697, #3758, #3856, #9272, #7291, #228, #14428, #11130, #6896, #2568, #8438, #7243, #15413, #10296, #6167, #7164, #12743 ) ) ;
#13313=CARTESIAN_POINT ( 'NONE',  ( 5.000000000000000000, -22.00000000000000000, 0.000000000000000000 ) ) ;
#13316=CARTESIAN_POINT ( 'NONE',  ( 1.846868145590736310, -22.87500000136559564, 4.458734124999999437 ) ) ;
#13320=CARTESIAN_POINT ( 'NONE',  ( -3.535533905932737309, -30.75000000273118772, -3.535533905932738197 ) ) ;
#13334=DIRECTION ( 'NONE',  ( 0.000000000000000000, 0.000000000000000000, -1.000000000000000000 ) ) ;
#13343=CARTESIAN_POINT ( 'NONE',  ( 24.26932219902320043, 40.00000000000000000, 5.999999999999992895 ) ) ;
#13346=SURFACE_STYLE_USAGE ( .BOTH. , #3491 ) ;
#13364=CARTESIAN_POINT ( 'NONE',  ( -5.000000000000000888, -22.68750000273119127, -2.071067811865475949 ) ) ;
#13365=CARTESIAN_POINT ( 'NONE',  ( 4.458734124999999437, -26.62500000136559564, -1.846868145590734978 ) ) ;
#13374=CARTESIAN_POINT ( 'NONE',  ( 4.458734124999999437, -23.68750000136559564, 0.000000000000000000 ) ) ;
#13375=CARTESIAN_POINT ( 'NONE',  ( -3.535533905932737309, -23.75000000273118772, -3.535533905932738197 ) ) ;
#13376=CARTESIAN_POINT ( 'NONE',  ( 2.071067811865461294, -29.93750000273118062, -5.000000000000014211 ) ) ;
#13381=CARTESIAN_POINT ( 'NONE',  ( 3.535533905932736864, -22.12500000000000000, 3.535533905932738641 ) ) ;
#13383=DIRECTION ( 'NONE',  ( -0.000000000000000000, 1.000000000000000000, -0.000000000000000000 ) ) ;
#13385=CARTESIAN_POINT ( 'NONE',  ( 1.846868145590735200, -25.25000000136559564, -4.458734125000000326 ) ) ;
#13387=ORIENTED_EDGE ( 'NONE', *, *, #6750, .T. ) ;
#13392=CARTESIAN_POINT ( 'NONE',  ( 3.152801135295366208, -26.56250000136559564, 3.152801135295367985 ) ) ;
#13395=CARTESIAN_POINT ( 'NONE',  ( -9.184850993605147944E-16, -28.25000000000000000, 5.000000000000000000 ) ) ;
#13397=EDGE_CURVE ( 'NONE', #8315, #12412, #10692, .T. ) ;
#13401=CARTESIAN_POINT ( 'NONE',  ( 3.152801135295366208, -22.81250000136559564, 3.152801135295367985 ) ) ;
#13403=CARTESIAN_POINT ( 'NONE',  ( 3.061616997868383141E-16, -31.75000000000000000, -5.000000000000000000 ) ) ;
#13410=EDGE_LOOP ( 'NONE', ( #10524, #6239, #14702 ) ) ;
#13426=CARTESIAN_POINT ( 'NONE',  ( 0.000000000000000000, -13.00000000000000178, 5.000000000000000000 ) ) ;
#13431=LINE ( 'NONE', #5778, #15213 ) ;
#13433=DIRECTION ( 'NONE',  ( 0.000000000000000000, 0.000000000000000000, 1.000000000000000000 ) ) ;
#13434=CARTESIAN_POINT ( 'NONE',  ( -1.846868145590737420, -26.00000000136560274, 4.458734124999997661 ) ) ;
#13435=CARTESIAN_POINT ( 'NONE',  ( -4.458734125000000326, -21.87500000136559208, 1.846868145590734089 ) ) ;
#13442=CARTESIAN_POINT ( 'NONE',  ( -3.152801135295367985, -22.06250000136559564, 3.152801135295367096 ) ) ;
#13445=DIRECTION ( 'NONE',  ( 1.000000000000000000, -0.000000000000000000, -1.239088197126290570E-16 ) ) ;
#13447=( BOUNDED_CURVE ( )  B_SPLINE_CURVE ( 2, ( #124, #8692, #13680, #1243, #5046, #6346, #11180, #8935, #14995 ),
 .UNSPECIFIED., .F., .F. ) 
 B_SPLINE_CURVE_WITH_KNOTS ( ( 3, 2, 2, 2, 3 ),
 ( 0.3750000000000000000, 0.3875000000000000111, 0.4000000000000000222, 0.4125000000000000333, 0.4250000000000000444 ),
 .UNSPECIFIED. ) 
 CURVE ( )  GEOMETRIC_REPRESENTATION_ITEM ( )  RATIONAL_B_SPLINE_CURVE ( ( 1.000000000000000000, 0.9238795325112867385, 1.000000000000000000, 0.9238795325112867385, 1.000000000000000000, 0.9238795325112867385, 1.000000000000000000, 0.9238795325112864054, 1.000000000000000444 ) ) 
 REPRESENTATION_ITEM ( '' )  );
#13448=CARTESIAN_POINT ( 'NONE',  ( -5.000000000000000888, -22.43749999999999645, 2.071067811865474617 ) ) ;
#13450=CARTESIAN_POINT ( 'NONE',  ( -2.071067811865482167, -27.68750000000000000, -4.999999999999992895 ) ) ;
#13451=CARTESIAN_POINT ( 'NONE',  ( -8.190561711645485556E-16, -27.68750000136559564, 4.458734124999999437 ) ) ;
#13455=VERTEX_POINT ( 'NONE', #2154 ) ;
#13457=DIRECTION ( 'NONE',  ( 0.000000000000000000, 0.000000000000000000, 1.000000000000000000 ) ) ;
#13458=CARTESIAN_POINT ( 'NONE',  ( 4.458734124999999437, -26.50000000136559208, 1.846868145590737864 ) ) ;
#13465=CYLINDRICAL_SURFACE ( 'NONE', #2806, 5.000000000000000000 ) ;
#13468=CARTESIAN_POINT ( 'NONE',  ( -4.458734125000000326, -22.25000000136559564, -1.846868145590735644 ) ) ;
#13471=CARTESIAN_POINT ( 'NONE',  ( -9.184850993605147944E-16, -30.37500000273118772, 5.000000000000000000 ) ) ;
#13474=CARTESIAN_POINT ( 'NONE',  ( 4.458734124999999437, -30.43750000136559564, 0.000000000000000000 ) ) ;
#13476=VERTEX_POINT ( 'NONE', #5879 ) ;
#13489=CARTESIAN_POINT ( 'NONE',  ( 35.00000000000000000, 40.00000000000000000, -2.650000000000001243 ) ) ;
#13490=CARTESIAN_POINT ( 'NONE',  ( -9.184850993605147944E-16, -22.25000000000000000, 5.000000000000000000 ) ) ;
#13492=FILL_AREA_STYLE ('',( #7306 ) ) ;
#13493=EDGE_CURVE ( 'NONE', #10237, #6755, #3653, .T. ) ;
#13499=VERTEX_POINT ( 'NONE', #5303 ) ;
#13501=AXIS2_PLACEMENT_3D ( 'NONE', #1772, #6719, #261 ) ;
#13506=CARTESIAN_POINT ( 'NONE',  ( -3.535533905932737309, -30.75000000273118772, -3.535533905932738197 ) ) ;
#13510=CARTESIAN_POINT ( 'NONE',  ( -2.071067811865478170, -22.43750000273118772, 5.000000000000000000 ) ) ;
#13511=CARTESIAN_POINT ( 'NONE',  ( 4.458734124999999437, -27.68750000136559564, 0.000000000000000000 ) ) ;
#13513=CARTESIAN_POINT ( 'NONE',  ( 0.000000000000000000, -20.00000000000000000, 0.000000000000000000 ) ) ;
#13517=ORIENTED_EDGE ( 'NONE', *, *, #9786, .T. ) ;
#13522=CARTESIAN_POINT ( 'NONE',  ( 4.458734124999999437, -22.75000000136559208, 1.846868145590737864 ) ) ;
#13525=CARTESIAN_POINT ( 'NONE',  ( -5.000000000000000000, -27.62500000273118772, -6.123233995736766282E-16 ) ) ;
#13533=CARTESIAN_POINT ( 'NONE',  ( 3.152801135295367541, -28.31250000136559564, -3.152801135295367541 ) ) ;
#13538=EDGE_LOOP ( 'NONE', ( #5099, #8134, #8551, #14211 ) ) ;
#13541=DIRECTION ( 'NONE',  ( -0.000000000000000000, 1.000000000000000000, -0.000000000000000000 ) ) ;
#13543=CARTESIAN_POINT ( 'NONE',  ( -4.458734124999999437, -22.93750000136559564, -5.460374474430324690E-16 ) ) ;
#13547=( BOUNDED_SURFACE ( )  B_SPLINE_SURFACE ( 1, 2, ( 
 ( #8280, #13170, #2106, #15779, #7050, #983, #13320, #1053, #3552, #5987, #11954, #5915, #13471, #6394, #12430, #6155, #7362, #7608, #7451, #12270, #10029, #9783, #14717, #12593, #2409, #5007, #13803, #3954, #4857, #13557, #11230, #9859, #14875, #8822, #12507, #5178, #6313, #11082, #2490, #1211, #11313, #1366, #15, #4933, #1449, #12357, #14791, #14964, #3638, #6066, #1289, #3711, #8898, #8583, #8658, #2739, #15039, #11150, #175, #10996, #15935, #263, #5094, #10107, #7696, #6234, #90, #2656, #9936, #3798, #8742, #13648, #2577, #7528, #3880, #13723, #10425, #13895, #2900, #10354, #15360, #12669, #12748, #5577, #15448, #12831, #1693, #7850, #5495, #4280, #14225, #3073, #6634, #11548, #1609, #9142, #14144, #9221, #1774, #4369, #11465, #500, #3149, #9066, #10514, #6722, #413, #5422, #10188, #11387, #8016, #8094, #12913, #10276, #1537, #11624, #15111, #1847, #6790, #11698, #6475, #9303, #14053, #2980, #653, #15281, #339, #574, #4195, #5252, #5337, #15204, #4032, #8983, #7934, #2824, #7778, #6550, #4118, #13968, #963, #7110, #2161, #10599, #9531, #1035, #15598, #3309, #10663, #12095, #10822, #6873, #11780, #2011, #10891, #14460, #3381, #13223, #15523, #733, #13297 ),
 ( #8261, #3531, #4673, #5889, #15762, #13153, #12014, #9597, #5658, #15832, #4515, #2088, #3452, #5805, #7195, #13073, #7033, #9376, #9672, #14534, #8405, #4752, #6960, #11933, #14610, #9450, #5970, #8332, #11861, #885, #4439, #14299, #2241, #12988, #1924, #5728, #3222, #8171, #808, #14381, #10742, #15679, #4593, #11292, #4988, #70, #13704, #8638, #8487, #3774, #13533, #13626, #7341, #12246, #7589, #7267, #12333, #4834, #10971, #14697, #13451, #9759, #12410, #2556, #7509, #6046, #9913, #12487, #11059, #14770, #6132, #1427, #1106, #15018, #15913, #7428, #243, #6374, #12168, #1468, #1346, #1187, #1270, #11208, #14942, #5161, #8720, #8563, #4913, #3618, #8800, #14853, #2392, #9838, #10003, #3692, #2468, #6293, #6215, #13385, #11131, #152, #10091, #5072, #3861, #2323, #2637, #9046, #14030, #10489, #8877, #7908, #2957, #9121, #1520, #476, #7994, #6531, #10253, #1592, #3047, #12572, #3933, #11370, #2880, #11680, #1827, #2716, #11445, #12808, #7761, #12728, #6701, #10405, #12895, #4174, #4010, #391, #321, #4256, #10336, #8961, #5231, #5476, #5311, #10167, #1751, #7674, #13783, #15179, #15090, #6772, #6457, #2805, #633, #5554, #13949, #11605, #13872, #12652, #9201 ) ),
 .UNSPECIFIED., .F., .F., .F. ) 
 B_SPLINE_SURFACE_WITH_KNOTS ( ( 2, 2 ),
 ( 3, 2, 2, 2, 2, 2, 2, 2, 2, 2, 2, 2, 2, 2, 2, 2, 2, 2, 2, 2, 2, 2, 2, 2, 2, 2, 2, 2, 2, 2, 2, 2, 2, 2, 2, 2, 2, 2, 2, 2, 2, 2, 2, 2, 2, 2, 2, 2, 2, 2, 2, 2, 2, 2, 2, 2, 2, 2, 2, 2, 2, 2, 2, 2, 2, 2, 2, 2, 2, 2, 2, 2, 2, 2, 2, 2, 2, 2, 2, 2, 3 ),
 ( 0.000000000000000000, 1.000000000000000000 ),
 ( 0.000000000000000000, 0.01250000000000000069, 0.02500000000000000139, 0.03749999999999999861, 0.05000000000000000278, 0.06250000000000000000, 0.07499999999999999722, 0.08749999999999999445, 0.1000000000000000056, 0.1125000000000000028, 0.1250000000000000000, 0.1375000000000000111, 0.1499999999999999944, 0.1625000000000000056, 0.1749999999999999889, 0.1875000000000000000, 0.2000000000000000111, 0.2124999999999999944, 0.2250000000000000056, 0.2374999999999999889, 0.2500000000000000000, 0.2625000000000000111, 0.2750000000000000222, 0.2874999999999999778, 0.2999999999999999889, 0.3125000000000000000, 0.3250000000000000111, 0.3375000000000000222, 0.3499999999999999778, 0.3624999999999999889, 0.3750000000000000000, 0.3875000000000000111, 0.4000000000000000222, 0.4124999999999999778, 0.4249999999999999889, 0.4375000000000000000, 0.4500000000000000111, 0.4625000000000000222, 0.4749999999999999778, 0.4874999999999999889, 0.5000000000000000000, 0.5124999999999999556, 0.5250000000000000222, 0.5374999999999999778, 0.5500000000000000444, 0.5625000000000000000, 0.5749999999999999556, 0.5875000000000000222, 0.5999999999999999778, 0.6125000000000000444, 0.6250000000000000000, 0.6374999999999999556, 0.6500000000000000222, 0.6624999999999999778, 0.6750000000000000444, 0.6875000000000000000, 0.6999999999999999556, 0.7125000000000000222, 0.7249999999999999778, 0.7375000000000000444, 0.7500000000000000000, 0.7624999999999999556, 0.7750000000000000222, 0.7874999999999999778, 0.8000000000000000444, 0.8125000000000000000, 0.8249999999999999556, 0.8375000000000000222, 0.8499999999999999778, 0.8625000000000000444, 0.8750000000000000000, 0.8874999999999999556, 0.9000000000000000222, 0.9124999999999999778, 0.9250000000000000444, 0.9375000000000000000, 0.9499999999999999556, 0.9625000000000000222, 0.9749999999999999778, 0.9875000000000000444, 1.000000000000000000 ),
 .UNSPECIFIED. ) 
 GEOMETRIC_REPRESENTATION_ITEM ( )  RATIONAL_B_SPLINE_SURFACE ( (
 ( 1.000000000000000000, 0.9238795325112867385, 1.000000000000000000, 0.9238795325112867385, 1.000000000000000000, 0.9238795325112867385, 1.000000000000000000, 0.9238795325112867385, 1.000000000000000000, 0.9238795325112867385, 1.000000000000000000, 0.9238795325112867385, 1.000000000000000000, 0.9238795325112867385, 1.000000000000000000, 0.9238795325112867385, 1.000000000000000000, 0.9238795325112867385, 1.000000000000000000, 0.9238795325112867385, 1.000000000000000000, 0.9238795325112867385, 1.000000000000000000, 0.9238795325112867385, 1.000000000000000000, 0.9238795325112867385, 1.000000000000000000, 0.9238795325112867385, 1.000000000000000000, 0.9238795325112867385, 1.000000000000000000, 0.9238795325112867385, 1.000000000000000000, 0.9238795325112867385, 1.000000000000000000, 0.9238795325112867385, 1.000000000000000000, 0.9238795325112867385, 1.000000000000000000, 0.9238795325112867385, 1.000000000000000000, 0.9238795325112867385, 1.000000000000000000, 0.9238795325112867385, 1.000000000000000000, 0.9238795325112867385, 1.000000000000000000, 0.9238795325112867385, 1.000000000000000000, 0.9238795325112867385, 1.000000000000000000, 0.9238795325112867385, 1.000000000000000000, 0.9238795325112867385, 1.000000000000000000, 0.9238795325112867385, 1.000000000000000000, 0.9238795325112867385, 1.000000000000000000, 0.9238795325112867385, 1.000000000000000000, 0.9238795325112867385, 1.000000000000000000, 0.9238795325112867385, 1.000000000000000000, 0.9238795325112867385, 1.000000000000000000, 0.9238795325112867385, 1.000000000000000000, 0.9238795325112867385, 1.000000000000000000, 0.9238795325112867385, 1.000000000000000000, 0.9238795325112867385, 1.000000000000000000, 0.9238795325112867385, 1.000000000000000000, 0.9238795325112867385, 1.000000000000000000, 0.9238795325112867385, 1.000000000000000000, 0.9238795325112867385, 1.000000000000000000, 0.9238795325112867385, 1.000000000000000000, 0.9238795325112867385, 1.000000000000000000, 0.9238795325112867385, 1.000000000000000000, 0.9238795325112867385, 1.000000000000000000, 0.9238795325112867385, 1.000000000000000000, 0.9238795325112867385, 1.000000000000000000, 0.9238795325112867385, 1.000000000000000000, 0.9238795325112867385, 1.000000000000000000, 0.9238795325112867385, 1.000000000000000000, 0.9238795325112867385, 1.000000000000000000, 0.9238795325112867385, 1.000000000000000000, 0.9238795325112867385, 1.000000000000000000, 0.9238795325112867385, 1.000000000000000000, 0.9238795325112867385, 1.000000000000000000, 0.9238795325112867385, 1.000000000000000000, 0.9238795325112867385, 1.000000000000000000, 0.9238795325112867385, 1.000000000000000000, 0.9238795325112867385, 1.000000000000000000, 0.9238795325112867385, 1.000000000000000000, 0.9238795325112867385, 1.000000000000000000, 0.9238795325112867385, 1.000000000000000000, 0.9238795325112867385, 1.000000000000000000, 0.9238795325112867385, 1.000000000000000000, 0.9238795325112867385, 1.000000000000000000, 0.9238795325112867385, 1.000000000000000000, 0.9238795325112867385, 1.000000000000000000, 0.9238795325112867385, 1.000000000000000000, 0.9238795325112867385, 1.000000000000000000, 0.9238795325112867385, 1.000000000000000000, 0.9238795325112867385, 1.000000000000000000, 0.9238795325112867385, 1.000000000000000000, 0.9238795325112867385, 1.000000000000000000, 0.9238795325112867385, 1.000000000000000000, 0.9238795325112867385, 1.000000000000000000, 0.9238795325112867385, 1.000000000000000000, 0.9238795325112867385, 1.000000000000000000, 0.9238795325112867385, 1.000000000000000000, 0.9238795325112867385, 1.000000000000000000, 0.9238795325112867385, 1.000000000000000000),
 ( 1.000000000000000000, 0.9238795325112867385, 1.000000000000000000, 0.9238795325112867385, 1.000000000000000000, 0.9238795325112867385, 1.000000000000000000, 0.9238795325112867385, 1.000000000000000000, 0.9238795325112867385, 1.000000000000000000, 0.9238795325112867385, 1.000000000000000000, 0.9238795325112867385, 1.000000000000000000, 0.9238795325112867385, 1.000000000000000000, 0.9238795325112867385, 1.000000000000000000, 0.9238795325112867385, 1.000000000000000000, 0.9238795325112867385, 1.000000000000000000, 0.9238795325112867385, 1.000000000000000000, 0.9238795325112867385, 1.000000000000000000, 0.9238795325112867385, 1.000000000000000000, 0.9238795325112867385, 1.000000000000000000, 0.9238795325112867385, 1.000000000000000000, 0.9238795325112867385, 1.000000000000000000, 0.9238795325112867385, 1.000000000000000000, 0.9238795325112867385, 1.000000000000000000, 0.9238795325112867385, 1.000000000000000000, 0.9238795325112867385, 1.000000000000000000, 0.9238795325112867385, 1.000000000000000000, 0.9238795325112867385, 1.000000000000000000, 0.9238795325112867385, 1.000000000000000000, 0.9238795325112867385, 1.000000000000000000, 0.9238795325112867385, 1.000000000000000000, 0.9238795325112867385, 1.000000000000000000, 0.9238795325112867385, 1.000000000000000000, 0.9238795325112867385, 1.000000000000000000, 0.9238795325112867385, 1.000000000000000000, 0.9238795325112867385, 1.000000000000000000, 0.9238795325112867385, 1.000000000000000000, 0.9238795325112867385, 1.000000000000000000, 0.9238795325112867385, 1.000000000000000000, 0.9238795325112867385, 1.000000000000000000, 0.9238795325112867385, 1.000000000000000000, 0.9238795325112867385, 1.000000000000000000, 0.9238795325112867385, 1.000000000000000000, 0.9238795325112867385, 1.000000000000000000, 0.9238795325112867385, 1.000000000000000000, 0.9238795325112867385, 1.000000000000000000, 0.9238795325112867385, 1.000000000000000000, 0.9238795325112867385, 1.000000000000000000, 0.9238795325112867385, 1.000000000000000000, 0.9238795325112867385, 1.000000000000000000, 0.9238795325112867385, 1.000000000000000000, 0.9238795325112867385, 1.000000000000000000, 0.9238795325112867385, 1.000000000000000000, 0.9238795325112867385, 1.000000000000000000, 0.9238795325112867385, 1.000000000000000000, 0.9238795325112867385, 1.000000000000000000, 0.9238795325112867385, 1.000000000000000000, 0.9238795325112867385, 1.000000000000000000, 0.9238795325112867385, 1.000000000000000000, 0.9238795325112867385, 1.000000000000000000, 0.9238795325112867385, 1.000000000000000000, 0.9238795325112867385, 1.000000000000000000, 0.9238795325112867385, 1.000000000000000000, 0.9238795325112867385, 1.000000000000000000, 0.9238795325112867385, 1.000000000000000000, 0.9238795325112867385, 1.000000000000000000, 0.9238795325112867385, 1.000000000000000000, 0.9238795325112867385, 1.000000000000000000, 0.9238795325112867385, 1.000000000000000000, 0.9238795325112867385, 1.000000000000000000, 0.9238795325112867385, 1.000000000000000000, 0.9238795325112867385, 1.000000000000000000, 0.9238795325112867385, 1.000000000000000000, 0.9238795325112867385, 1.000000000000000000, 0.9238795325112867385, 1.000000000000000000, 0.9238795325112867385, 1.000000000000000000, 0.9238795325112867385, 1.000000000000000000, 0.9238795325112867385, 1.000000000000000000, 0.9238795325112867385, 1.000000000000000000, 0.9238795325112867385, 1.000000000000000000, 0.9238795325112867385, 1.000000000000000000, 0.9238795325112867385, 1.000000000000000000, 0.9238795325112867385, 1.000000000000000000, 0.9238795325112867385, 1.000000000000000000, 0.9238795325112867385, 1.000000000000000000) ) ) 
 REPRESENTATION_ITEM ( '' )  SURFACE ( )  );
#13548=VECTOR ( 'NONE', #324, 1000.000000000000000 ) ;
#13553=CARTESIAN_POINT ( 'NONE',  ( -4.458734124999999437, -25.18750000136559564, -5.460374474430324690E-16 ) ) ;
#13555=ADVANCED_FACE ( 'NONE', ( #1657 ), #5389, .T. ) ;
#13557=CARTESIAN_POINT ( 'NONE',  ( 2.071067811865476394, -29.31250000273118417, 5.000000000000000000 ) ) ;
#13559=CARTESIAN_POINT ( 'NONE',  ( -3.152801135295367096, -31.06250000136559564, -3.152801135295367541 ) ) ;
#13567=CARTESIAN_POINT ( 'NONE',  ( 4.729367062499999719, -21.84375000068279604, 0.000000000000000000 ) ) ;
#13573=EDGE_CURVE ( 'NONE', #6357, #2056, #2629, .T. ) ;
#13577=CIRCLE ( 'NONE', #14377, 5.999999999999991118 ) ;
#13586=VERTEX_POINT ( 'NONE', #1337 ) ;
#13595=ADVANCED_FACE ( 'NONE', ( #11197 ), #143, .T. ) ;
#13600=LINE ( 'NONE', #13929, #6942 ) ;
#13601=CARTESIAN_POINT ( 'NONE',  ( 4.458734124999999437, -24.68750000136559564, 0.000000000000000000 ) ) ;
#13603=CARTESIAN_POINT ( 'NONE',  ( -4.458734125000000326, -23.87500000136559564, 1.846868145590734089 ) ) ;
#13612=CARTESIAN_POINT ( 'NONE',  ( -4.458734124999999437, -24.18750000136559564, -5.460374474430324690E-16 ) ) ;
#13626=CARTESIAN_POINT ( 'NONE',  ( 1.846868145590735200, -28.25000000136559208, -4.458734125000000326 ) ) ;
#13631=ORIENTED_EDGE ( 'NONE', *, *, #14088, .T. ) ;
#13635=CARTESIAN_POINT ( 'NONE',  ( 3.152801135295367541, -26.31250000136559564, -3.152801135295367541 ) ) ;
#13644=EDGE_CURVE ( 'NONE', #7371, #9203, #2708, .T. ) ;
#13645=CARTESIAN_POINT ( 'NONE',  ( 3.535533905932736864, -31.12500000000000000, 3.535533905932738641 ) ) ;
#13648=CARTESIAN_POINT ( 'NONE',  ( -5.000000000000000888, -26.68750000273119127, -2.071067811865475949 ) ) ;
#13650=CARTESIAN_POINT ( 'NONE',  ( -4.458734124999999437, -30.00000000136559919, -1.846868145590735644 ) ) ;
#13660=CARTESIAN_POINT ( 'NONE',  ( -4.458734124999999437, -31.18750000136559564, -5.460374474430324690E-16 ) ) ;
#13665=CARTESIAN_POINT ( 'NONE',  ( 3.535533905932738197, -23.87500000000000000, -3.535533905932738197 ) ) ;
#13669=VERTEX_POINT ( 'NONE', #7665 ) ;
#13671=CARTESIAN_POINT ( 'NONE',  ( 4.458734124999999437, -21.43750000136559208, 0.000000000000000000 ) ) ;
#13679=PRODUCT_DEFINITION_CONTEXT ( 'detailed design', #12991, 'design' ) ;
#13680=CARTESIAN_POINT ( 'NONE',  ( 3.535533905932736864, -27.25000000273118772, 3.535533905932738641 ) ) ;
#13682=CARTESIAN_POINT ( 'NONE',  ( 6.000000000000000000, -13.00000000000000178, -1.500000000000000000 ) ) ;
#13684=CARTESIAN_POINT ( 'NONE',  ( 2.730187237215162345E-16, -25.43750000136559564, -4.458734124999999437 ) ) ;
#13685=ORIENTED_EDGE ( 'NONE', *, *, #1043, .T. ) ;
#13689=EDGE_LOOP ( 'NONE', ( #12903, #1172, #15941, #14363, #1414 ) ) ;
#13693=CARTESIAN_POINT ( 'NONE',  ( -3.152801135295367096, -22.31250000136559564, -3.152801135295367541 ) ) ;
#13704=CARTESIAN_POINT ( 'NONE',  ( 3.152801135295366208, -28.56250000136559564, 3.152801135295367985 ) ) ;
#13710=CARTESIAN_POINT ( 'NONE',  ( 0.000000000000000000, -20.00000000000000000, 5.000000000000000000 ) ) ;
#13711=CARTESIAN_POINT ( 'NONE',  ( -4.458734124999999437, -23.93750000136559564, -5.460374474430324690E-16 ) ) ;
#13712=ADVANCED_FACE ( 'NONE', ( #4334, #10478 ), #7900, .T. ) ;
#13720=CARTESIAN_POINT ( 'NONE',  ( 2.071067811865475505, -31.81250000000000000, -5.000000000000000888 ) ) ;
#13721=CARTESIAN_POINT ( 'NONE',  ( 35.00000000000000000, 37.00000000000000000, -2.649999999999994582 ) ) ;
#13723=CARTESIAN_POINT ( 'NONE',  ( -2.071067811865478170, -26.43750000273119127, 5.000000000000000000 ) ) ;
#13725=CARTESIAN_POINT ( 'NONE',  ( 1.846868145590736310, -28.62500000136559564, 4.458734124999997661 ) ) ;
#13727=ORIENTED_EDGE ( 'NONE', *, *, #14920, .T. ) ;
#13729=VECTOR ( 'NONE', #6175, 1000.000000000000000 ) ;
#13737=AXIS2_PLACEMENT_3D ( 'NONE', #2820, #491, #4113 ) ;
#13743=( BOUNDED_CURVE ( )  B_SPLINE_CURVE ( 2, ( #6206, #7498, #9902, #1335, #6281 ),
 .UNSPECIFIED., .F., .F. ) 
 B_SPLINE_CURVE_WITH_KNOTS ( ( 3, 2, 3 ),
 ( 0.000000000000000000, 0.01250000000000001110, 0.02500000000000002220 ),
 .UNSPECIFIED. ) 
 CURVE ( )  GEOMETRIC_REPRESENTATION_ITEM ( )  RATIONAL_B_SPLINE_CURVE ( ( 1.000000000000000000, 0.9238795325112867385, 1.000000000000000000, 0.9238795325112866275, 1.000000000000000222 ) ) 
 REPRESENTATION_ITEM ( '' )  );
#13760=CARTESIAN_POINT ( 'NONE',  ( 3.061616997868383141E-16, -23.75000000000000000, -5.000000000000000000 ) ) ;
#13770=VERTEX_POINT ( 'NONE', #10639 ) ;
#13783=CARTESIAN_POINT ( 'NONE',  ( 2.730187237215162345E-16, -22.18750000136559564, -4.458734124999999437 ) ) ;
#13789=CARTESIAN_POINT ( 'NONE',  ( 1.846868145590735200, -31.50000000136559564, -4.458734125000000326 ) ) ;
#13790=CARTESIAN_POINT ( 'NONE',  ( 0.000000000000000000, -20.00000000000000000, 5.000000000000000000 ) ) ;
#13798=CARTESIAN_POINT ( 'NONE',  ( -9.184850993605147944E-16, -28.25000000000000000, 5.000000000000000000 ) ) ;
#13803=CARTESIAN_POINT ( 'NONE',  ( -3.535533905932738641, -29.50000000273118417, 3.535533905932737309 ) ) ;
#13806=CARTESIAN_POINT ( 'NONE',  ( 1.846868145590736310, -30.62500000136559564, 4.458734124999997661 ) ) ;
#13814=ORIENTED_EDGE ( 'NONE', *, *, #7812, .F. ) ;
#13819=CARTESIAN_POINT ( 'NONE',  ( -3.535533905932737309, -31.62500000000000000, -3.535533905932738197 ) ) ;
#13837=ORIENTED_EDGE ( 'NONE', *, *, #12564, .F. ) ;
#13853=ORIENTED_EDGE ( 'NONE', *, *, #6935, .F. ) ;
#13863=DIRECTION ( 'NONE',  ( -1.000000000000000000, 0.000000000000000000, 0.000000000000000000 ) ) ;
#13872=CARTESIAN_POINT ( 'NONE',  ( 3.152801135295366208, -21.56250000136559208, 3.152801135295367985 ) ) ;
#13874=EDGE_LOOP ( 'NONE', ( #11866, #9841, #8842, #7633 ) ) ;
#13878=ORIENTED_EDGE ( 'NONE', *, *, #5802, .T. ) ;
#13879=CARTESIAN_POINT ( 'NONE',  ( 3.152801135295367541, -30.56250000136559564, -3.152801135295367541 ) ) ;
#13884=EDGE_CURVE ( 'NONE', #3455, #8368, #13194, .T. ) ;
#13891=CARTESIAN_POINT ( 'NONE',  ( 3.061616997868383141E-16, -28.75000000000000000, -5.000000000000000000 ) ) ;
#13895=CARTESIAN_POINT ( 'NONE',  ( 2.071067811865476394, -26.31250000273118417, 5.000000000000000000 ) ) ;
#13898=CARTESIAN_POINT ( 'NONE',  ( -1.846868145590734756, -27.12500000136559564, -4.458734124999999437 ) ) ;
#13906=DIRECTION ( 'NONE',  ( 0.000000000000000000, 0.000000000000000000, 1.000000000000000000 ) ) ;
#13907=ADVANCED_FACE ( 'NONE', ( #1237 ), #5860, .T. ) ;
#13911=CARTESIAN_POINT ( 'NONE',  ( -4.458734125000000326, -30.25000000136559564, -1.846868145590735644 ) ) ;
#13916=CYLINDRICAL_SURFACE ( 'NONE', #741, 5.000000000000000000 ) ;
#13919=CARTESIAN_POINT ( 'NONE',  ( -35.00000000000000000, 37.00000000000000000, 0.000000000000000000 ) ) ;
#13923=EDGE_CURVE ( 'NONE', #8374, #8967, #403, .T. ) ;
#13926=CARTESIAN_POINT ( 'NONE',  ( 0.000000000000000000, -20.00000000000000000, 0.000000000000000000 ) ) ;
#13929=CARTESIAN_POINT ( 'NONE',  ( 6.000000000000000000, -13.00000000000000178, 1.500000000000000000 ) ) ;
#13930=CARTESIAN_POINT ( 'NONE',  ( 1.846868145590736310, -22.87500000136559564, 4.458734124999997661 ) ) ;
#13931=ORIENTED_EDGE ( 'NONE', *, *, #13213, .F. ) ;
#13938=EDGE_CURVE ( 'NONE', #3489, #3157, #9179, .T. ) ;
#13945=CYLINDRICAL_SURFACE ( 'NONE', #2803, 5.000000000000000000 ) ;
#13947=DIRECTION ( 'NONE',  ( 0.000000000000000000, 0.000000000000000000, 1.000000000000000000 ) ) ;
#13949=CARTESIAN_POINT ( 'NONE',  ( -8.190561711645485556E-16, -21.68750000136559208, 4.458734124999999437 ) ) ;
#13955=ORIENTED_EDGE ( 'NONE', *, *, #6738, .T. ) ;
#13956=CARTESIAN_POINT ( 'NONE',  ( -3.152801135295367096, -29.31250000136559564, -3.152801135295367541 ) ) ;
#13964=CARTESIAN_POINT ( 'NONE',  ( -5.000000000000000888, -30.56250000000000000, -2.071067811865475949 ) ) ;
#13967=DIRECTION ( 'NONE',  ( 1.239088197126290570E-16, -0.000000000000000000, 1.000000000000000000 ) ) ;
#13968=CARTESIAN_POINT ( 'NONE',  ( -2.071067811865478170, -22.43750000273119127, 5.000000000000000000 ) ) ;
#13970=CARTESIAN_POINT ( 'NONE',  ( 1.846868145590735200, -25.25000000136559564, -4.458734124999999437 ) ) ;
#13973=VERTEX_POINT ( 'NONE', #13426 ) ;
#13983=CARTESIAN_POINT ( 'NONE',  ( -1.846868145590737420, -31.00000000136559564, 4.458734124999999437 ) ) ;
#14009=ORIENTED_EDGE ( 'NONE', *, *, #7999, .F. ) ;
#14012=VECTOR ( 'NONE', #12431, 1000.000000000000000 ) ;
#14013=CARTESIAN_POINT ( 'NONE',  ( -2.071067811865463959, -26.43750000273118772, 5.000000000000013323 ) ) ;
#14019=DIRECTION ( 'NONE',  ( -0.000000000000000000, 1.000000000000000000, -0.000000000000000000 ) ) ;
#14030=CARTESIAN_POINT ( 'NONE',  ( -8.190561711645485556E-16, -24.68750000136559564, 4.458734124999999437 ) ) ;
#14037=VERTEX_POINT ( 'NONE', #8772 ) ;
#14040=CARTESIAN_POINT ( 'NONE',  ( 4.458734124999999437, -30.68750000136559564, 0.000000000000000000 ) ) ;
#14049=CARTESIAN_POINT ( 'NONE',  ( -3.535533905932737309, -27.62500000000000000, -3.535533905932738197 ) ) ;
#14052=CARTESIAN_POINT ( 'NONE',  ( 0.000000000000000000, -13.00000000000000178, 0.000000000000000000 ) ) ;
#14053=CARTESIAN_POINT ( 'NONE',  ( -3.535533905932738641, -23.50000000273118772, 3.535533905932737309 ) ) ;
#14054=EDGE_CURVE ( 'NONE', #9435, #11992, #2606, .T. ) ;
#14057=CARTESIAN_POINT ( 'NONE',  ( -4.458734125000000326, -24.87500000136559564, 1.846868145590734089 ) ) ;
#14065=ORIENTED_EDGE ( 'NONE', *, *, #15753, .T. ) ;
#14072=CARTESIAN_POINT ( 'NONE',  ( -8.190561711645485556E-16, -26.93750000136559564, 4.458734124999999437 ) ) ;
#14082=CARTESIAN_POINT ( 'NONE',  ( -4.458734124999999437, -27.93750000136559564, -5.460374474430324690E-16 ) ) ;
#14088=EDGE_CURVE ( 'NONE', #15165, #11995, #8203, .T. ) ;
#14099=CARTESIAN_POINT ( 'NONE',  ( -3.152801135295367096, -22.31250000136559564, -3.152801135295367541 ) ) ;
#14100=VERTEX_POINT ( 'NONE', #1958 ) ;
#14105=AXIS2_PLACEMENT_3D ( 'NONE', #14652, #5931, #2356 ) ;
#14108=DIRECTION ( 'NONE',  ( -0.000000000000000000, 1.000000000000000000, -0.000000000000000000 ) ) ;
#14113=CARTESIAN_POINT ( 'NONE',  ( -9.184850993605147944E-16, -25.37500000273118417, 5.000000000000000000 ) ) ;
#14129=CARTESIAN_POINT ( 'NONE',  ( 4.458734124999999437, -30.75000000136559564, 1.846868145590737864 ) ) ;
#14139=CARTESIAN_POINT ( 'NONE',  ( 5.000000000000000888, -24.93750000000000355, -2.071067811865475505 ) ) ;
#14144=CARTESIAN_POINT ( 'NONE',  ( 5.000000000000000000, -25.12500000273118417, 0.000000000000000000 ) ) ;
#14147=CARTESIAN_POINT ( 'NONE',  ( -3.152801135295367096, -28.06250000136559564, -3.152801135295367541 ) ) ;
#14156=ORIENTED_EDGE ( 'NONE', *, *, #499, .T. ) ;
#14162=CARTESIAN_POINT ( 'NONE',  ( -5.000000000000000888, -31.43750000000000000, 2.071067811865474617 ) ) ;
#14163=CARTESIAN_POINT ( 'NONE',  ( -4.458734124999999437, -29.18750000136559564, -5.460374474430324690E-16 ) ) ;
#14165=CARTESIAN_POINT ( 'NONE',  ( -9.184850993605147944E-16, -24.25000000000000000, 5.000000000000000000 ) ) ;
#14179=VECTOR ( 'NONE', #3867, 1000.000000000000000 ) ;
#14195=CARTESIAN_POINT ( 'NONE',  ( 2.071067811865461294, -22.93750000273118417, -5.000000000000014211 ) ) ;
#14200=CARTESIAN_POINT ( 'NONE',  ( -2.071067811865460850, -25.68750000000000355, -5.000000000000014211 ) ) ;
#14203=CARTESIAN_POINT ( 'NONE',  ( 4.769696007084728073, -13.00000000000000178, 1.500000000000000000 ) ) ;
#14205=CARTESIAN_POINT ( 'NONE',  ( 4.458734124999999437, -29.68750000136559208, 0.000000000000000000 ) ) ;
#14207=ORIENTED_EDGE ( 'NONE', *, *, #5298, .F. ) ;
#14209=EDGE_CURVE ( 'NONE', #15920, #2123, #11808, .T. ) ;
#14211=ORIENTED_EDGE ( 'NONE', *, *, #3443, .F. ) ;
#14215=CARTESIAN_POINT ( 'NONE',  ( -3.152801135295367985, -29.06250000136559564, 3.152801135295367096 ) ) ;
#14218=CARTESIAN_POINT ( 'NONE',  ( -2.071067811865478170, -28.31250000000000000, 5.000000000000000000 ) ) ;
#14222=CARTESIAN_POINT ( 'NONE',  ( 2.071067811865476394, -24.18750000000000355, 5.000000000000000000 ) ) ;
#14225=CARTESIAN_POINT ( 'NONE',  ( -3.535533905932738641, -25.50000000273118417, 3.535533905932737309 ) ) ;
#14227=CARTESIAN_POINT ( 'NONE',  ( -4.458734124999999437, -26.93750000136559564, -5.460374474430324690E-16 ) ) ;
#14238=CARTESIAN_POINT ( 'NONE',  ( -4.458734125000001214, -27.12500000136559564, 1.846868145590734089 ) ) ;
#14247=EDGE_CURVE ( 'NONE', #10561, #4719, #15887, .T. ) ;
#14256=( NAMED_UNIT ( * ) PLANE_ANGLE_UNIT ( ) SI_UNIT ( $, .RADIAN. ) );
#14257=DIRECTION ( 'NONE',  ( 0.000000000000000000, 1.000000000000000000, 0.000000000000000000 ) ) ;
#14262=DIRECTION ( 'NONE',  ( 0.000000000000000000, -1.000000000000000000, 0.000000000000000000 ) ) ;
#14268=CARTESIAN_POINT ( 'NONE',  ( -5.000000000000000888, -30.43750000000000355, 2.071067811865474617 ) ) ;
#14277=LINE ( 'NONE', #9280, #4739 ) ;
#14278=VECTOR ( 'NONE', #727, 1000.000000000000000 ) ;
#14280=CARTESIAN_POINT ( 'NONE',  ( 2.730187237215162345E-16, -28.43750000136559564, -4.458734124999999437 ) ) ;
#14287=CARTESIAN_POINT ( 'NONE',  ( -3.152801135295367096, -27.31250000136559564, -3.152801135295367541 ) ) ;
#14295=CARTESIAN_POINT ( 'NONE',  ( -2.071067811865478170, -26.31250000000000355, 5.000000000000000000 ) ) ;
#14299=CARTESIAN_POINT ( 'NONE',  ( 4.458734124999999437, -29.50000000136559564, 1.846868145590737864 ) ) ;
#14307=CARTESIAN_POINT ( 'NONE',  ( -9.184850993605147944E-16, -29.37500000273118417, 5.000000000000000000 ) ) ;
#14312=CARTESIAN_POINT ( 'NONE',  ( 1.846868145590735200, -27.50000000136559208, -4.458734125000000326 ) ) ;
#14316=CARTESIAN_POINT ( 'NONE',  ( 2.071067811865485275, -31.18749999999999645, 4.999999999999989342 ) ) ;
#14319=CARTESIAN_POINT ( 'NONE',  ( 6.123233995736766282E-16, -11.00000000000000178, -5.000000000000000000 ) ) ;
#14328=EDGE_CURVE ( 'NONE', #8368, #5406, #8625, .T. ) ;
#14350=CIRCLE ( 'NONE', #8669, 25.00000000000000000 ) ;
#14353=CYLINDRICAL_SURFACE ( 'NONE', #12802, 5.000000000000000000 ) ;
#14356=CARTESIAN_POINT ( 'NONE',  ( 35.00000000000000000, 40.00000000000000000, -8.572527594031472993E-15 ) ) ;
#14358=CARTESIAN_POINT ( 'NONE',  ( 2.071067811865505259, -25.31250000273118062, 4.999999999999970690 ) ) ;
#14359=CARTESIAN_POINT ( 'NONE',  ( -4.458734124999999437, -30.18750000136559564, -5.460374474430324690E-16 ) ) ;
#14363=ORIENTED_EDGE ( 'NONE', *, *, #9169, .F. ) ;
#14365=CIRCLE ( 'NONE', #9464, 25.00000000000000000 ) ;
#14366=CARTESIAN_POINT ( 'NONE',  ( 2.730187237215162345E-16, -26.43750000136559564, -4.458734124999999437 ) ) ;
#14369=LINE ( 'NONE', #15669, #4284 ) ;
#14375=AXIS2_PLACEMENT_3D ( 'NONE', #7579, #14931, #3850 ) ;
#14376=CARTESIAN_POINT ( 'NONE',  ( -5.000000000000000000, -26.50000000000000355, -6.123233995736766282E-16 ) ) ;
#14377=AXIS2_PLACEMENT_3D ( 'NONE', #13919, #11340, #11256 ) ;
#14381=CARTESIAN_POINT ( 'NONE',  ( -4.458734125000000326, -29.00000000136559564, -1.846868145590735644 ) ) ;
#14390=CARTESIAN_POINT ( 'NONE',  ( -3.152801135295367985, -26.81250000136559564, 3.152801135295367096 ) ) ;
#14391=EDGE_CURVE ( 'NONE', #4663, #12836, #11907, .T. ) ;
#14392=FACE_OUTER_BOUND ( 'NONE', #1951, .T. ) ;
#14398=CARTESIAN_POINT ( 'NONE',  ( 1.846868145590735200, -28.50000000136559564, -4.458734125000000326 ) ) ;
#14401=FACE_OUTER_BOUND ( 'NONE', #8295, .T. ) ;
#14403=DIRECTION ( 'NONE',  ( 0.000000000000000000, 1.000000000000000000, 0.000000000000000000 ) ) ;
#14413=CARTESIAN_POINT ( 'NONE',  ( -5.000000000000000888, -26.43750000000000711, 2.071067811865474617 ) ) ;
#14419=CARTESIAN_POINT ( 'NONE',  ( -9.184850993605147944E-16, -22.37500000273118417, 5.000000000000000000 ) ) ;
#14422=CARTESIAN_POINT ( 'NONE',  ( 24.26932219902320043, 40.00000000000000000, -5.999999999999989342 ) ) ;
#14426=CARTESIAN_POINT ( 'NONE',  ( 35.00000000000000000, 40.00000000000000000, 5.999999999999991118 ) ) ;
#14427=ORIENTED_EDGE ( 'NONE', *, *, #8832, .F. ) ;
#14428=ADVANCED_FACE ( 'NONE', ( #14401 ), #13547, .T. ) ;
#14435=CARTESIAN_POINT ( 'NONE',  ( 35.00000000000000000, 37.00000000000000000, -5.999999999999991118 ) ) ;
#14441=CARTESIAN_POINT ( 'NONE',  ( 1.846868145590735200, -28.50000000136559564, -4.458734124999999437 ) ) ;
#14445=ADVANCED_FACE ( 'NONE', ( #556 ), #7832, .T. ) ;
#14451=CARTESIAN_POINT ( 'NONE',  ( -1.846868145590734756, -26.37500000136559564, -4.458734125000000326 ) ) ;
#14452=CARTESIAN_POINT ( 'NONE',  ( -2.071067811865475061, -23.81250000273118772, -5.000000000000000888 ) ) ;
#14455=LINE ( 'NONE', #10420, #14278 ) ;
#14456=CARTESIAN_POINT ( 'NONE',  ( 5.000000000000000000, -22.00000000000000000, 0.000000000000000000 ) ) ;
#14458=CARTESIAN_POINT ( 'NONE',  ( -3.535533905932737309, -21.75000000273118772, -3.535533905932738197 ) ) ;
#14460=CARTESIAN_POINT ( 'NONE',  ( -2.071067811865478170, -21.43750000273119127, 5.000000000000000000 ) ) ;
#14463=ORIENTED_EDGE ( 'NONE', *, *, #8743, .F. ) ;
#14465=CARTESIAN_POINT ( 'NONE',  ( 0.000000000000000000, 20.00000000000000000, 25.00000000000000000 ) ) ;
#14466=EDGE_CURVE ( 'NONE', #9203, #6666, #3048, .T. ) ;
#14467=CARTESIAN_POINT ( 'NONE',  ( 3.152801135295367541, -27.31250000136559564, -3.152801135295367541 ) ) ;
#14469=ORIENTED_EDGE ( 'NONE', *, *, #3722, .F. ) ;
#14472=DIRECTION ( 'NONE',  ( 0.000000000000000000, 0.000000000000000000, 1.000000000000000000 ) ) ;
#14473=CARTESIAN_POINT ( 'NONE',  ( 4.458734124999999437, -23.75000000136559208, 1.846868145590737864 ) ) ;
#14485=CARTESIAN_POINT ( 'NONE',  ( 0.000000000000000000, -13.00000000000000178, 0.000000000000000000 ) ) ;
#14488=EDGE_CURVE ( 'NONE', #12412, #8728, #8857, .T. ) ;
#14494=CARTESIAN_POINT ( 'NONE',  ( -2.071067811865450192, -22.31250000000000000, 5.000000000000028422 ) ) ;
#14496=VERTEX_POINT ( 'NONE', #7969 ) ;
#14502=DIRECTION ( 'NONE',  ( 0.000000000000000000, 0.000000000000000000, 1.000000000000000000 ) ) ;
#14503=EDGE_CURVE ( 'NONE', #349, #9262, #3988, .T. ) ;
#14511=CARTESIAN_POINT ( 'NONE',  ( 2.730187237215162345E-16, -29.43750000136559208, -4.458734124999999437 ) ) ;
#14513=ORIENTED_EDGE ( 'NONE', *, *, #1683, .F. ) ;
#14516=VECTOR ( 'NONE', #4314, 1000.000000000000000 ) ;
#14517=ORIENTED_EDGE ( 'NONE', *, *, #7117, .T. ) ;
#14520=CARTESIAN_POINT ( 'NONE',  ( 4.458734125000000326, -28.62500000136559919, -1.846868145590734978 ) ) ;
#14521=CARTESIAN_POINT ( 'NONE',  ( -2.071067811865478170, -23.43750000273119127, 5.000000000000000000 ) ) ;
#14529=ADVANCED_FACE ( 'NONE', ( #11351 ), #301, .F. ) ;
#14530=CARTESIAN_POINT ( 'NONE',  ( 4.458734124999999437, -31.43750000136559564, 0.000000000000000000 ) ) ;
#14534=CARTESIAN_POINT ( 'NONE',  ( 1.846868145590735200, -30.25000000136559564, -4.458734125000000326 ) ) ;
#14535=VERTEX_POINT ( 'NONE', #1573 ) ;
#14540=CARTESIAN_POINT ( 'NONE',  ( -4.458734125000000326, -30.00000000136559564, -1.846868145590735644 ) ) ;
#14548=CARTESIAN_POINT ( 'NONE',  ( -4.458734125000000326, -24.25000000136559564, -1.846868145590735644 ) ) ;
#14553=ORIENTED_EDGE ( 'NONE', *, *, #13397, .T. ) ;
#14556=DIRECTION ( 'NONE',  ( 0.000000000000000000, 0.000000000000000000, 1.000000000000000000 ) ) ;
#14558=EDGE_CURVE ( 'NONE', #12414, #379, #15236, .T. ) ;
#14571=ORIENTED_EDGE ( 'NONE', *, *, #1483, .F. ) ;
#14587=CARTESIAN_POINT ( 'NONE',  ( 1.846868145590736310, -24.87500000136559564, 4.458734124999997661 ) ) ;
#14596=CARTESIAN_POINT ( 'NONE',  ( 1.846868145590736310, -21.87500000136559208, 4.458734124999999437 ) ) ;
#14605=CARTESIAN_POINT ( 'NONE',  ( -9.184850993605147944E-16, -23.25000000000000000, 5.000000000000000000 ) ) ;
#14610=CARTESIAN_POINT ( 'NONE',  ( -4.458734124999999437, -29.93750000136559564, -5.460374474430324690E-16 ) ) ;
#14617=ORIENTED_EDGE ( 'NONE', *, *, #1683, .T. ) ;
#14618=PLANE ( 'NONE',  #4378 ) ;
#14619=CARTESIAN_POINT ( 'NONE',  ( -8.190561711645485556E-16, -23.68750000136559564, 4.458734124999999437 ) ) ;
#14631=CARTESIAN_POINT ( 'NONE',  ( -8.190561711645485556E-16, -21.93750000136559208, 4.458734124999999437 ) ) ;
#14638=CARTESIAN_POINT ( 'NONE',  ( -35.00000000000000000, 37.00000000000000000, -5.999999999999991118 ) ) ;
#14652=CARTESIAN_POINT ( 'NONE',  ( 0.000000000000000000, -32.00000000000000000, 0.000000000000000000 ) ) ;
#14654=CARTESIAN_POINT ( 'NONE',  ( 2.071067811865476394, -22.31250000273118417, 5.000000000000000000 ) ) ;
#14656=CARTESIAN_POINT ( 'NONE',  ( -5.000000000000000000, -22.50000000000000000, -6.123233995736766282E-16 ) ) ;
#14666=CARTESIAN_POINT ( 'NONE',  ( -5.000000000000000888, -29.56250000000000355, -2.071067811865475949 ) ) ;
#14669=DIRECTION ( 'NONE',  ( -0.000000000000000000, -1.000000000000000000, -0.000000000000000000 ) ) ;
#14674=CARTESIAN_POINT ( 'NONE',  ( 4.458734124999997661, -24.75000000136559564, 1.846868145590737864 ) ) ;
#14678=VERTEX_POINT ( 'NONE', #5690 ) ;
#14685=CARTESIAN_POINT ( 'NONE',  ( -4.458734125000000326, -24.25000000136559564, -1.846868145590735644 ) ) ;
#14686=FACE_OUTER_BOUND ( 'NONE', #12574, .T. ) ;
#14697=CARTESIAN_POINT ( 'NONE',  ( -1.846868145590737420, -27.75000000136559564, 4.458734124999999437 ) ) ;
#14701=EDGE_LOOP ( 'NONE', ( #7063, #14065, #4819, #5409 ) ) ;
#14702=ORIENTED_EDGE ( 'NONE', *, *, #5522, .F. ) ;
#14704=CARTESIAN_POINT ( 'NONE',  ( 4.458734125000000326, -25.37500000136559919, -1.846868145590734978 ) ) ;
#14707=CARTESIAN_POINT ( 'NONE',  ( 0.000000000000000000, 40.00000000000000000, 0.000000000000000000 ) ) ;
#14712=CARTESIAN_POINT ( 'NONE',  ( -1.846868145590737420, -23.00000000136559564, 4.458734124999999437 ) ) ;
#14717=CARTESIAN_POINT ( 'NONE',  ( -3.535533905932737309, -29.75000000273118417, -3.535533905932738197 ) ) ;
#14720=CARTESIAN_POINT ( 'NONE',  ( 5.000000000000000000, -25.06250000000000000, 2.071067811865478614 ) ) ;
#14729=EDGE_CURVE ( 'NONE', #9634, #2989, #13109, .T. ) ;
#14735=CARTESIAN_POINT ( 'NONE',  ( 3.061616997868383141E-16, -22.75000000000000000, -4.999999999999999112 ) ) ;
#14737=CARTESIAN_POINT ( 'NONE',  ( 6.000000000000000000, -20.00000000000000000, -1.500000000000000000 ) ) ;
#14742=CARTESIAN_POINT ( 'NONE',  ( 0.000000000000000000, -13.00000000000000178, -1.500000000000000000 ) ) ;
#14746=CARTESIAN_POINT ( 'NONE',  ( 3.061616997868383141E-16, -30.87500000273118772, -5.000000000000000000 ) ) ;
#14749=CARTESIAN_POINT ( 'NONE',  ( -4.458734124999999437, -24.25000000136559564, -1.846868145590735644 ) ) ;
#14750=CARTESIAN_POINT ( 'NONE',  ( 4.458734124999999437, -23.43750000136559564, 0.000000000000000000 ) ) ;
#14758=CARTESIAN_POINT ( 'NONE',  ( -8.190561711645485556E-16, -22.93750000136559564, 4.458734124999999437 ) ) ;
#14759=CARTESIAN_POINT ( 'NONE',  ( 0.000000000000000000, 37.00000000000000000, 0.000000000000000000 ) ) ;
#14764=FACE_OUTER_BOUND ( 'NONE', #8271, .T. ) ;
#14766=CARTESIAN_POINT ( 'NONE',  ( 2.071067811865475505, -22.81250000000000000, -5.000000000000000888 ) ) ;
#14770=CARTESIAN_POINT ( 'NONE',  ( -1.846868145590734756, -27.12500000136559564, -4.458734125000000326 ) ) ;
#14776=DIRECTION ( 'NONE',  ( 0.000000000000000000, 1.000000000000000000, 0.000000000000000000 ) ) ;
#14777=CARTESIAN_POINT ( 'NONE',  ( -1.846868145590734756, -23.12500000136559564, -4.458734125000000326 ) ) ;
#14787=CARTESIAN_POINT ( 'NONE',  ( -4.458734125000001214, -24.12500000136559919, 1.846868145590734089 ) ) ;
#14791=CARTESIAN_POINT ( 'NONE',  ( 3.535533905932736864, -28.25000000273118772, 3.535533905932738641 ) ) ;
#14794=CARTESIAN_POINT ( 'NONE',  ( 3.061616997868383141E-16, -23.87500000273118772, -5.000000000000000000 ) ) ;
#14799=( BOUNDED_CURVE ( )  B_SPLINE_CURVE ( 2, ( #341, #7698, #9861, #8746, #5181, #10109, #3800, #6396, #14794 ),
 .UNSPECIFIED., .F., .F. ) 
 B_SPLINE_CURVE_WITH_KNOTS ( ( 3, 2, 2, 2, 3 ),
 ( 0.6749999999999999334, 0.6874999999999998890, 0.6999999999999999556, 0.7125000000000000222, 0.7249999999999999778 ),
 .UNSPECIFIED. ) 
 CURVE ( )  GEOMETRIC_REPRESENTATION_ITEM ( )  RATIONAL_B_SPLINE_CURVE ( ( 1.000000000000000666, 0.9238795325112860723, 1.000000000000000000, 0.9238795325112867385, 1.000000000000000000, 0.9238795325112867385, 1.000000000000000000, 0.9238795325112867385, 1.000000000000000000 ) ) 
 REPRESENTATION_ITEM ( '' )  );
#14804=CARTESIAN_POINT ( 'NONE',  ( 3.061616997868383141E-16, -25.87500000273118417, -5.000000000000000000 ) ) ;
#14809=CYLINDRICAL_SURFACE ( 'NONE', #10550, 5.000000000000000000 ) ;
#14826=CARTESIAN_POINT ( 'NONE',  ( 6.000000000000000000, -13.00000000000000178, 1.500000000000000000 ) ) ;
#14831=CARTESIAN_POINT ( 'NONE',  ( -1.846868145590734756, -26.37500000136559564, -4.458734124999999437 ) ) ;
#14834=CARTESIAN_POINT ( 'NONE',  ( -3.152801135295367096, -24.06250000136559564, -3.152801135295367541 ) ) ;
#14836=CARTESIAN_POINT ( 'NONE',  ( 35.00000000000000000, 40.00000000000000000, 5.999999999999991118 ) ) ;
#14838=ORIENTED_EDGE ( 'NONE', *, *, #11102, .T. ) ;
#14841=CARTESIAN_POINT ( 'NONE',  ( 1.846868145590735200, -24.50000000136559564, -4.458734125000000326 ) ) ;
#14848=CARTESIAN_POINT ( 'NONE',  ( 0.000000000000000000, -13.00000000000000178, 0.000000000000000000 ) ) ;
#14852=DIRECTION ( 'NONE',  ( 1.000000000000000000, 0.000000000000000000, 0.000000000000000000 ) ) ;
#14853=CARTESIAN_POINT ( 'NONE',  ( -1.846868145590737420, -25.75000000136559564, 4.458734124999999437 ) ) ;
#14860=AXIS2_PLACEMENT_3D ( 'NONE', #10522, #4603, #6799 ) ;
#14862=CARTESIAN_POINT ( 'NONE',  ( 4.458734124999999437, -25.43750000136559564, 0.000000000000000000 ) ) ;
#14871=CARTESIAN_POINT ( 'NONE',  ( -5.000000000000000888, -28.56250000000000000, -2.071067811865475949 ) ) ;
#14875=CARTESIAN_POINT ( 'NONE',  ( 5.000000000000000000, -29.12500000273118772, 0.000000000000000000 ) ) ;
#14877=CARTESIAN_POINT ( 'NONE',  ( -4.458734125000000326, -29.87500000136559564, 1.846868145590734089 ) ) ;
#14886=ORIENTED_EDGE ( 'NONE', *, *, #15093, .F. ) ;
#14888=LINE ( 'NONE', #13567, #1459 ) ;
#14901=( BOUNDED_CURVE ( )  B_SPLINE_CURVE ( 2, ( #13760, #12704, #2694, #6349, #5209, #4150, #9096, #6509, #10144 ),
 .UNSPECIFIED., .F., .F. ) 
 B_SPLINE_CURVE_WITH_KNOTS ( ( 3, 2, 2, 2, 3 ),
 ( 0.8250000000000000666, 0.8375000000000001332, 0.8500000000000000888, 0.8625000000000000444, 0.8750000000000000000 ),
 .UNSPECIFIED. ) 
 CURVE ( )  GEOMETRIC_REPRESENTATION_ITEM ( )  RATIONAL_B_SPLINE_CURVE ( ( 0.9999999999999993339, 0.9238795325112874046, 1.000000000000000000, 0.9238795325112867385, 1.000000000000000000, 0.9238795325112867385, 1.000000000000000000, 0.9238795325112867385, 1.000000000000000000 ) ) 
 REPRESENTATION_ITEM ( '' )  );
#14902=CARTESIAN_POINT ( 'NONE',  ( 0.000000000000000000, -20.00000000000000000, 0.000000000000000000 ) ) ;
#14912=VECTOR ( 'NONE', #12592, 1000.000000000000000 ) ;
#14918=CARTESIAN_POINT ( 'NONE',  ( 2.071067811865462183, -28.31250000273118772, 5.000000000000013323 ) ) ;
#14919=CARTESIAN_POINT ( 'NONE',  ( -4.458734124999999437, -27.18750000136559564, -5.460374474430324690E-16 ) ) ;
#14920=EDGE_CURVE ( 'NONE', #13455, #14678, #7899, .T. ) ;
#14929=CARTESIAN_POINT ( 'NONE',  ( 1.846868145590736310, -23.87500000136559564, 4.458734124999999437 ) ) ;
#14931=DIRECTION ( 'NONE',  ( -0.000000000000000000, 1.000000000000000000, -0.000000000000000000 ) ) ;
#14935=CARTESIAN_POINT ( 'NONE',  ( 3.061616997868383141E-16, -25.75000000000000355, -5.000000000000000000 ) ) ;
#14942=CARTESIAN_POINT ( 'NONE',  ( 2.730187237215162345E-16, -26.18750000136559564, -4.458734124999999437 ) ) ;
#14949=ORIENTED_EDGE ( 'NONE', *, *, #1440, .F. ) ;
#14952=CARTESIAN_POINT ( 'NONE',  ( -3.152801135295367096, -24.06250000136559564, -3.152801135295367541 ) ) ;
#14953=DIRECTION ( 'NONE',  ( 0.000000000000000000, 0.000000000000000000, -1.000000000000000000 ) ) ;
#14954=VERTEX_POINT ( 'NONE', #6726 ) ;
#14961=CARTESIAN_POINT ( 'NONE',  ( -2.071067811865475061, -28.68750000000000711, -5.000000000000000888 ) ) ;
#14964=CARTESIAN_POINT ( 'NONE',  ( 5.000000000000000000, -28.18750000273119127, 2.071067811865478614 ) ) ;
#14966=CARTESIAN_POINT ( 'NONE',  ( 0.000000000000000000, -13.00000000000000178, 1.500000000000000000 ) ) ;
#14967=CARTESIAN_POINT ( 'NONE',  ( -1.846868145590734756, -30.12500000136559564, -4.458734124999999437 ) ) ;
#14969=ORIENTED_EDGE ( 'NONE', *, *, #11945, .F. ) ;
#14977=CARTESIAN_POINT ( 'NONE',  ( -3.152801135295367985, -31.06250000136559564, 3.152801135295367096 ) ) ;
#14984=ORIENTED_EDGE ( 'NONE', *, *, #14729, .T. ) ;
#14992=CARTESIAN_POINT ( 'NONE',  ( -2.071067811865457742, -28.81250000273119127, -5.000000000000019540 ) ) ;
#14995=CARTESIAN_POINT ( 'NONE',  ( 3.061616997868383141E-16, -26.87500000273118772, -5.000000000000000000 ) ) ;
#14999=DIRECTION ( 'NONE',  ( 0.000000000000000000, -1.000000000000000000, 0.000000000000000000 ) ) ;
#15000=VERTEX_POINT ( 'NONE', #2326 ) ;
#15007=FACE_OUTER_BOUND ( 'NONE', #3321, .T. ) ;
#15011=CARTESIAN_POINT ( 'NONE',  ( 2.071067811865490160, -25.81250000000000355, -4.999999999999985789 ) ) ;
#15013=DIRECTION ( 'NONE',  ( -0.000000000000000000, 1.000000000000000000, -0.000000000000000000 ) ) ;
#15018=CARTESIAN_POINT ( 'NONE',  ( -4.458734125000001214, -26.87500000136559208, 1.846868145590734089 ) ) ;
#15024=CARTESIAN_POINT ( 'NONE',  ( -4.458734125000001214, -21.87500000136559208, 1.846868145590734089 ) ) ;
#15026=EDGE_LOOP ( 'NONE', ( #12280, #11135, #1867, #1111 ) ) ;
#15036=CARTESIAN_POINT ( 'NONE',  ( -5.000000000000000888, -28.43750000000000355, 2.071067811865474617 ) ) ;
#15039=CARTESIAN_POINT ( 'NONE',  ( -5.000000000000000000, -27.62500000273118772, -6.123233995736766282E-16 ) ) ;
#15041=CARTESIAN_POINT ( 'NONE',  ( -3.152801135295367096, -29.06250000136559564, -3.152801135295367541 ) ) ;
#15044=ORIENTED_EDGE ( 'NONE', *, *, #2364, .F. ) ;
#15051=DIRECTION ( 'NONE',  ( 0.000000000000000000, 0.000000000000000000, 1.000000000000000000 ) ) ;
#15052=CARTESIAN_POINT ( 'NONE',  ( -4.458734125000001214, -30.12500000136559208, 1.846868145590734089 ) ) ;
#15057=ORIENTED_EDGE ( 'NONE', *, *, #9216, .F. ) ;
#15064=DIRECTION ( 'NONE',  ( 0.000000000000000000, 1.000000000000000000, 0.000000000000000000 ) ) ;
#15065=CARTESIAN_POINT ( 'NONE',  ( 5.000000000000000000, -21.18750000273119127, 2.071067811865478614 ) ) ;
#15066=CARTESIAN_POINT ( 'NONE',  ( -2.071067811865477726, -30.81250000273118062, -4.999999999999996447 ) ) ;
#15070=CARTESIAN_POINT ( 'NONE',  ( -4.458734125000000326, -23.12500000136559564, 1.846868145590734089 ) ) ;
#15072=CARTESIAN_POINT ( 'NONE',  ( 0.000000000000000000, -11.00000000000000178, 0.000000000000000000 ) ) ;
#15081=DIRECTION ( 'NONE',  ( -0.000000000000000000, 1.000000000000000000, -0.000000000000000000 ) ) ;
#15085=DIRECTION ( 'NONE',  ( 1.000000000000000000, 0.000000000000000000, 0.000000000000000000 ) ) ;
#15090=CARTESIAN_POINT ( 'NONE',  ( -3.152801135295367096, -22.06250000136559564, -3.152801135295367541 ) ) ;
#15093=EDGE_CURVE ( 'NONE', #8967, #6357, #2976, .T. ) ;
#15098=AXIS2_PLACEMENT_3D ( 'NONE', #8940, #2782, #7740 ) ;
#15099=CARTESIAN_POINT ( 'NONE',  ( -3.152801135295367096, -22.06250000136559564, -3.152801135295367541 ) ) ;
#15107=CARTESIAN_POINT ( 'NONE',  ( -2.071067811865478170, -31.31250000000000000, 5.000000000000000000 ) ) ;
#15111=CARTESIAN_POINT ( 'NONE',  ( 3.061616997868383141E-16, -23.87500000273118772, -5.000000000000000000 ) ) ;
#15113=CARTESIAN_POINT ( 'NONE',  ( 3.152801135295367541, -26.31250000136559564, -3.152801135295367541 ) ) ;
#15115=ORIENTED_EDGE ( 'NONE', *, *, #12797, .T. ) ;
#15119=ORIENTED_EDGE ( 'NONE', *, *, #2112, .T. ) ;
#15131=VECTOR ( 'NONE', #222, 1000.000000000000000 ) ;
#15134=VERTEX_POINT ( 'NONE', #4837 ) ;
#15135=VECTOR ( 'NONE', #10655, 1000.000000000000000 ) ;
#15148=VECTOR ( 'NONE', #8755, 1000.000000000000000 ) ;
#15149=PLANE ( 'NONE',  #5135 ) ;
#15150=VECTOR ( 'NONE', #1655, 1000.000000000000000 ) ;
#15156=CARTESIAN_POINT ( 'NONE',  ( 6.123233995736766282E-16, -20.00000000000000000, -5.000000000000000000 ) ) ;
#15157=ORIENTED_EDGE ( 'NONE', *, *, #14558, .F. ) ;
#15158=DIRECTION ( 'NONE',  ( 0.000000000000000000, 0.000000000000000000, -1.000000000000000000 ) ) ;
#15161=CARTESIAN_POINT ( 'NONE',  ( 0.000000000000000000, -20.00000000000000000, 5.000000000000000000 ) ) ;
#15165=VERTEX_POINT ( 'NONE', #10007 ) ;
#15169=VECTOR ( 'NONE', #11030, 1000.000000000000000 ) ;
#15172=DIRECTION ( 'NONE',  ( -0.000000000000000000, -1.000000000000000000, -0.000000000000000000 ) ) ;
#15174=VECTOR ( 'NONE', #9336, 1000.000000000000000 ) ;
#15179=CARTESIAN_POINT ( 'NONE',  ( -1.846868145590734756, -22.12500000136559564, -4.458734125000000326 ) ) ;
#15185=ORIENTED_EDGE ( 'NONE', *, *, #3213, .T. ) ;
#15188=CARTESIAN_POINT ( 'NONE',  ( 4.458734124999999437, -31.68750000136559564, 0.000000000000000000 ) ) ;
#15199=CARTESIAN_POINT ( 'NONE',  ( -3.535533905932737309, -31.62500000000000000, -3.535533905932738197 ) ) ;
#15201=CARTESIAN_POINT ( 'NONE',  ( 3.061616997868383141E-16, -21.87500000273118772, -5.000000000000000000 ) ) ;
#15203=CARTESIAN_POINT ( 'NONE',  ( -24.26932219902319687, 40.00000000000000000, 5.999999999999998224 ) ) ;
#15204=CARTESIAN_POINT ( 'NONE',  ( 2.071067811865475505, -22.93750000273119127, -5.000000000000000888 ) ) ;
#15206=AXIS2_PLACEMENT_3D ( 'NONE', #6327, #11402, #10205 ) ;
#15207=CARTESIAN_POINT ( 'NONE',  ( 1.846868145590736310, -27.62500000136559564, 4.458734124999997661 ) ) ;
#15209=ORIENTED_EDGE ( 'NONE', *, *, #9108, .F. ) ;
#15213=VECTOR ( 'NONE', #14669, 1000.000000000000000 ) ;
#15227=EDGE_LOOP ( 'NONE', ( #1433, #3493, #5196, #14463 ) ) ;
#15232=EDGE_CURVE ( 'NONE', #11992, #5212, #8666, .T. ) ;
#15236=( BOUNDED_CURVE ( )  B_SPLINE_CURVE ( 2, ( #8129, #5763, #10916, #14720, #3557, #6912, #9787, #13026, #614 ),
 .UNSPECIFIED., .F., .F. ) 
 B_SPLINE_CURVE_WITH_KNOTS ( ( 3, 2, 2, 2, 3 ),
 ( 0.6749999999999999334, 0.6874999999999998890, 0.6999999999999999556, 0.7125000000000000222, 0.7249999999999999778 ),
 .UNSPECIFIED. ) 
 CURVE ( )  GEOMETRIC_REPRESENTATION_ITEM ( )  RATIONAL_B_SPLINE_CURVE ( ( 1.000000000000000666, 0.9238795325112860723, 1.000000000000000000, 0.9238795325112867385, 1.000000000000000000, 0.9238795325112867385, 1.000000000000000000, 0.9238795325112867385, 1.000000000000000000 ) ) 
 REPRESENTATION_ITEM ( '' )  );
#15238=CARTESIAN_POINT ( 'NONE',  ( -3.535533905932738641, -28.50000000273118772, 3.535533905932737309 ) ) ;
#15243=CARTESIAN_POINT ( 'NONE',  ( 3.152801135295366208, -22.81250000136559564, 3.152801135295367985 ) ) ;
#15245=PLANE ( 'NONE',  #7440 ) ;
#15254=CARTESIAN_POINT ( 'NONE',  ( 0.000000000000000000, -20.00000000000000000, 0.000000000000000000 ) ) ;
#15260=CARTESIAN_POINT ( 'NONE',  ( -35.00000000000000000, 40.00000000000000000, -5.999999999999991118 ) ) ;
#15267=VERTEX_POINT ( 'NONE', #2395 ) ;
#15269=CARTESIAN_POINT ( 'NONE',  ( -1.846868145590737420, -21.75000000136559564, 4.458734124999999437 ) ) ;
#15277=CARTESIAN_POINT ( 'NONE',  ( 5.000000000000000888, -26.93750000000000711, -2.071067811865475505 ) ) ;
#15281=CARTESIAN_POINT ( 'NONE',  ( 2.071067811865476394, -23.31250000273118772, 5.000000000000000000 ) ) ;
#15283=CARTESIAN_POINT ( 'NONE',  ( -4.458734124999999437, -24.93750000136559564, -5.460374474430324690E-16 ) ) ;
#15295=FACE_OUTER_BOUND ( 'NONE', #13285, .T. ) ;
#15297=CARTESIAN_POINT ( 'NONE',  ( 3.152801135295366208, -30.81250000136559564, 3.152801135295367985 ) ) ;
#15305=CARTESIAN_POINT ( 'NONE',  ( 2.730187237215162345E-16, -27.18750000136559564, -4.458734124999999437 ) ) ;
#15306=EDGE_CURVE ( 'NONE', #11064, #3993, #933, .T. ) ;
#15318=CARTESIAN_POINT ( 'NONE',  ( 4.458734124999999437, -23.68750000136559564, 0.000000000000000000 ) ) ;
#15324=EDGE_CURVE ( 'NONE', #4537, #10561, #12898, .T. ) ;
#15325=ORIENTED_EDGE ( 'NONE', *, *, #9216, .T. ) ;
#15337=CARTESIAN_POINT ( 'NONE',  ( 3.535533905932738197, -22.87500000000000000, -3.535533905932738197 ) ) ;
#15348=CARTESIAN_POINT ( 'NONE',  ( -4.458734125000001214, -30.12500000136559208, 1.846868145590734089 ) ) ;
#15356=CARTESIAN_POINT ( 'NONE',  ( 2.071067811865476394, -25.18750000000000000, 5.000000000000000000 ) ) ;
#15360=CARTESIAN_POINT ( 'NONE',  ( 5.000000000000000000, -26.12500000273118417, 0.000000000000000000 ) ) ;
#15363=CARTESIAN_POINT ( 'NONE',  ( 4.458734124999999437, -28.43750000136559564, 0.000000000000000000 ) ) ;
#15366=ORIENTED_EDGE ( 'NONE', *, *, #227, .T. ) ;
#15370=CARTESIAN_POINT ( 'NONE',  ( 3.535533905932736864, -29.25000000273118772, 3.535533905932738641 ) ) ;
#15374=AXIS2_PLACEMENT_3D ( 'NONE', #1667, #6609, #11523 ) ;
#15375=DIRECTION ( 'NONE',  ( -0.000000000000000000, 1.000000000000000000, -0.000000000000000000 ) ) ;
#15376=CARTESIAN_POINT ( 'NONE',  ( 1.846868145590736310, -28.87500000136559564, 4.458734124999999437 ) ) ;
#15381=ORIENTED_EDGE ( 'NONE', *, *, #13493, .F. ) ;
#15387=ORIENTED_EDGE ( 'NONE', *, *, #5522, .T. ) ;
#15394=CIRCLE ( 'NONE', #13298, 5.000000000000000000 ) ;
#15413=ADVANCED_FACE ( 'NONE', ( #6775 ), #10258, .T. ) ;
#15414=CARTESIAN_POINT ( 'NONE',  ( 3.061616997868383141E-16, -25.87500000273118417, -5.000000000000000000 ) ) ;
#15422=CARTESIAN_POINT ( 'NONE',  ( 0.000000000000000000, 40.00000000000000000, 25.00000000000000000 ) ) ;
#15423=CARTESIAN_POINT ( 'NONE',  ( -1.846868145590737420, -29.00000000136559564, 4.458734124999997661 ) ) ;
#15432=CARTESIAN_POINT ( 'NONE',  ( -4.458734125000001214, -27.12500000136559564, 1.846868145590734089 ) ) ;
#15434=AXIS2_PLACEMENT_3D ( 'NONE', #1397, #7562, #122 ) ;
#15443=CARTESIAN_POINT ( 'NONE',  ( -2.071067811865478170, -24.31250000000000000, 5.000000000000000000 ) ) ;
#15445=CARTESIAN_POINT ( 'NONE',  ( -9.184850993605147944E-16, -21.37500000273118772, 5.000000000000000000 ) ) ;
#15448=CARTESIAN_POINT ( 'NONE',  ( 3.061616997868383141E-16, -25.87500000273118417, -5.000000000000000000 ) ) ;
#15451=CARTESIAN_POINT ( 'NONE',  ( 4.458734124999997661, -27.50000000136559564, 1.846868145590737864 ) ) ;
#15457=ORIENTED_EDGE ( 'NONE', *, *, #6840, .F. ) ;
#15459=VECTOR ( 'NONE', #14852, 1000.000000000000000 ) ;
#15463=CARTESIAN_POINT ( 'NONE',  ( 3.152801135295366208, -25.81250000136559564, 3.152801135295367985 ) ) ;
#15485=DIRECTION ( 'NONE',  ( 0.000000000000000000, 1.000000000000000000, 0.000000000000000000 ) ) ;
#15490=ORIENTED_EDGE ( 'NONE', *, *, #4846, .F. ) ;
#15494=DIRECTION ( 'NONE',  ( 0.000000000000000000, 0.000000000000000000, 1.000000000000000000 ) ) ;
#15499=CARTESIAN_POINT ( 'NONE',  ( -2.071067811865492381, -25.31250000000000000, 4.999999999999985789 ) ) ;
#15502=DIRECTION ( 'NONE',  ( 0.000000000000000000, 0.000000000000000000, -1.000000000000000000 ) ) ;
#15504=CARTESIAN_POINT ( 'NONE',  ( -4.458734124999999437, -31.18750000136559564, -5.460374474430324690E-16 ) ) ;
#15512=CARTESIAN_POINT ( 'NONE',  ( -8.190561711645485556E-16, -28.93750000136559564, 4.458734124999999437 ) ) ;
#15514=EDGE_CURVE ( 'NONE', #2381, #15134, #12777, .T. ) ;
#15519=CARTESIAN_POINT ( 'NONE',  ( -5.000000000000000888, -24.56250000000000000, -2.071067811865475949 ) ) ;
#15523=CARTESIAN_POINT ( 'NONE',  ( 3.535533905932736864, -21.25000000273118772, 3.535533905932738641 ) ) ;
#15524=ORIENTED_EDGE ( 'NONE', *, *, #7812, .T. ) ;
#15525=CARTESIAN_POINT ( 'NONE',  ( -8.190561711645485556E-16, -21.68750000136559208, 4.458734124999999437 ) ) ;
#15531=CARTESIAN_POINT ( 'NONE',  ( 3.061616997868383141E-16, -28.87500000273118772, -5.000000000000000000 ) ) ;
#15538=CARTESIAN_POINT ( 'NONE',  ( -4.458734125000000326, -28.25000000136559208, -1.846868145590735644 ) ) ;
#15564=CARTESIAN_POINT ( 'NONE',  ( 2.071067811865461294, -26.81249999999999289, -5.000000000000014211 ) ) ;
#15568=CARTESIAN_POINT ( 'NONE',  ( 0.000000000000000000, -20.00000000000000000, 0.000000000000000000 ) ) ;
#15579=CARTESIAN_POINT ( 'NONE',  ( -3.152801135295367096, -30.31250000136559564, -3.152801135295367541 ) ) ;
#15581=ORIENTED_EDGE ( 'NONE', *, *, #9103, .T. ) ;
#15586=CARTESIAN_POINT ( 'NONE',  ( -8.190561711645485556E-16, -25.93750000136559564, 4.458734124999999437 ) ) ;
#15587=LINE ( 'NONE', #5717, #5332 ) ;
#15589=CARTESIAN_POINT ( 'NONE',  ( 3.061616997868383141E-16, -29.75000000000000000, -5.000000000000000000 ) ) ;
#15592=CARTESIAN_POINT ( 'NONE',  ( 3.535533905932736864, -27.12500000000000000, 3.535533905932738641 ) ) ;
#15597=EDGE_CURVE ( 'NONE', #15267, #12836, #9984, .T. ) ;
#15598=CARTESIAN_POINT ( 'NONE',  ( 3.535533905932738197, -22.00000000273118772, -3.535533905932738197 ) ) ;
#15600=CARTESIAN_POINT ( 'NONE',  ( -8.190561711645485556E-16, -22.68750000136559564, 4.458734124999999437 ) ) ;
#15604=CARTESIAN_POINT ( 'NONE',  ( 3.061616997868383141E-16, -22.75000000000000000, -5.000000000000000000 ) ) ;
#15605=CARTESIAN_POINT ( 'NONE',  ( 1.846868145590736310, -27.62500000136559564, 4.458734124999999437 ) ) ;
#15608=ORIENTED_EDGE ( 'NONE', *, *, #7478, .T. ) ;
#15609=CARTESIAN_POINT ( 'NONE',  ( -5.000000000000000000, -24.62500000273118417, -6.123233995736766282E-16 ) ) ;
#15611=CARTESIAN_POINT ( 'NONE',  ( 3.152801135295367541, -28.56250000136559564, -3.152801135295367541 ) ) ;
#15613=DIRECTION ( 'NONE',  ( 0.000000000000000000, -1.000000000000000000, 0.000000000000000000 ) ) ;
#15618=AXIS2_PLACEMENT_3D ( 'NONE', #3852, #8951, #13863 ) ;
#15620=ORIENTED_EDGE ( 'NONE', *, *, #846, .T. ) ;
#15645=EDGE_LOOP ( 'NONE', ( #15325, #1562, #14207, #5056 ) ) ;
#15651=CARTESIAN_POINT ( 'NONE',  ( 35.00000000000000000, 37.00000000000000000, -8.572527594031472993E-15 ) ) ;
#15652=EDGE_CURVE ( 'NONE', #7272, #9435, #5315, .T. ) ;
#15653=DIRECTION ( 'NONE',  ( 0.000000000000000000, 1.000000000000000000, 0.000000000000000000 ) ) ;
#15656=CARTESIAN_POINT ( 'NONE',  ( 3.152801135295366208, -29.81250000136559208, 3.152801135295367985 ) ) ;
#15657=( BOUNDED_CURVE ( )  B_SPLINE_CURVE ( 2, ( #6252, #3655, #2427, #108, #5027, #9957, #13665, #2595, #7549 ),
 .UNSPECIFIED., .F., .F. ) 
 B_SPLINE_CURVE_WITH_KNOTS ( ( 3, 2, 2, 2, 3 ),
 ( 0.7750000000000000222, 0.7874999999999999778, 0.8000000000000000444, 0.8125000000000001110, 0.8250000000000000666 ),
 .UNSPECIFIED. ) 
 CURVE ( )  GEOMETRIC_REPRESENTATION_ITEM ( )  RATIONAL_B_SPLINE_CURVE ( ( 1.000000000000000000, 0.9238795325112867385, 1.000000000000000000, 0.9238795325112867385, 1.000000000000000000, 0.9238795325112867385, 1.000000000000000000, 0.9238795325112860723, 1.000000000000000666 ) ) 
 REPRESENTATION_ITEM ( '' )  );
#15660=( GEOMETRIC_REPRESENTATION_CONTEXT ( 3 ) GLOBAL_UNCERTAINTY_ASSIGNED_CONTEXT ( ( #607 ) ) GLOBAL_UNIT_ASSIGNED_CONTEXT ( ( #5032, #9719, #3583 ) ) REPRESENTATION_CONTEXT ( 'NONE', 'WORKASPACE' ) );
#15667=CARTESIAN_POINT ( 'NONE',  ( 2.730187237215162345E-16, -25.43750000136559564, -4.458734124999999437 ) ) ;
#15669=CARTESIAN_POINT ( 'NONE',  ( -35.00000000000000000, 37.00000000000000000, 6.000000000000000000 ) ) ;
#15674=AXIS2_PLACEMENT_3D ( 'NONE', #1788, #7706, #13906 ) ;
#15679=CARTESIAN_POINT ( 'NONE',  ( -4.458734125000001214, -28.87500000136559564, 1.846868145590734089 ) ) ;
#15681=CARTESIAN_POINT ( 'NONE',  ( 4.458734124999997661, -21.50000000136559208, 1.846868145590737864 ) ) ;
#15687=CARTESIAN_POINT ( 'NONE',  ( 4.458734125000000326, -28.37500000136559564, -1.846868145590734978 ) ) ;
#15693=DIRECTION ( 'NONE',  ( -0.000000000000000000, 1.000000000000000000, -0.000000000000000000 ) ) ;
#15695=AXIS2_PLACEMENT_3D ( 'NONE', #14356, #3285, #8232 ) ;
#15697=CARTESIAN_POINT ( 'NONE',  ( -1.846868145590737420, -24.00000000136559564, 4.458734124999999437 ) ) ;
#15703=ORIENTED_EDGE ( 'NONE', *, *, #11477, .F. ) ;
#15713=CARTESIAN_POINT ( 'NONE',  ( -5.000000000000000000, -26.50000000000000355, -6.123233995736766282E-16 ) ) ;
#15722=CARTESIAN_POINT ( 'NONE',  ( 3.535533905932738197, -22.00000000273118772, -3.535533905932738197 ) ) ;
#15731=ORIENTED_EDGE ( 'NONE', *, *, #11368, .F. ) ;
#15732=EDGE_CURVE ( 'NONE', #6357, #10561, #9897, .T. ) ;
#15733=AXIS2_PLACEMENT_3D ( 'NONE', #14052, #12830, #3308 ) ;
#15736=EDGE_CURVE ( 'NONE', #6755, #14037, #7744, .T. ) ;
#15740=DIRECTION ( 'NONE',  ( 0.000000000000000000, 0.000000000000000000, 1.000000000000000000 ) ) ;
#15742=CARTESIAN_POINT ( 'NONE',  ( 4.458734124999997661, -29.75000000136559564, 1.846868145590737864 ) ) ;
#15751=CARTESIAN_POINT ( 'NONE',  ( 1.846868145590735200, -28.50000000136559564, -4.458734125000000326 ) ) ;
#15753=EDGE_CURVE ( 'NONE', #3455, #2036, #7494, .T. ) ;
#15760=CARTESIAN_POINT ( 'NONE',  ( -3.535533905932738641, -21.50000000273118772, 3.535533905932737309 ) ) ;
#15762=CARTESIAN_POINT ( 'NONE',  ( 2.730187237215162345E-16, -31.18750000136559564, -4.458734124999999437 ) ) ;
#15763=ORIENTED_EDGE ( 'NONE', *, *, #14503, .F. ) ;
#15769=CARTESIAN_POINT ( 'NONE',  ( 1.846868145590735200, -29.25000000136559564, -4.458734125000000326 ) ) ;
#15773=CARTESIAN_POINT ( 'NONE',  ( -35.00000000000000000, 37.00000000000000000, -5.999999999999991118 ) ) ;
#15776=CARTESIAN_POINT ( 'NONE',  ( -4.458734124999999437, -23.18750000136559564, -5.460374474430324690E-16 ) ) ;
#15779=CARTESIAN_POINT ( 'NONE',  ( 2.071067811865475505, -30.93750000273118772, -5.000000000000000888 ) ) ;
#15803=ORIENTED_EDGE ( 'NONE', *, *, #1953, .F. ) ;
#15809=CARTESIAN_POINT ( 'NONE',  ( -5.000000000000000000, -29.62500000273118417, -6.123233995736766282E-16 ) ) ;
#15813=CARTESIAN_POINT ( 'NONE',  ( 3.152801135295366208, -24.81250000136559564, 3.152801135295367985 ) ) ;
#15819=VERTEX_POINT ( 'NONE', #305 ) ;
#15823=DIRECTION ( 'NONE',  ( -0.000000000000000000, -1.000000000000000000, -0.000000000000000000 ) ) ;
#15831=CARTESIAN_POINT ( 'NONE',  ( -5.000000000000000000, -27.50000000000000000, -6.123233995736766282E-16 ) ) ;
#15832=CARTESIAN_POINT ( 'NONE',  ( -4.458734125000001214, -30.87500000136559564, 1.846868145590734089 ) ) ;
#15836=ORIENTED_EDGE ( 'NONE', *, *, #1439, .F. ) ;
#15841=CARTESIAN_POINT ( 'NONE',  ( 1.846868145590735200, -28.25000000136559208, -4.458734125000000326 ) ) ;
#15847=DIRECTION ( 'NONE',  ( 0.000000000000000000, -1.000000000000000000, 0.000000000000000000 ) ) ;
#15849=DIRECTION ( 'NONE',  ( 0.000000000000000000, 0.000000000000000000, 1.000000000000000000 ) ) ;
#15850=CARTESIAN_POINT ( 'NONE',  ( -4.458734125000001214, -22.12500000136559564, 1.846868145590734089 ) ) ;
#15866=CARTESIAN_POINT ( 'NONE',  ( 3.535533905932736864, -28.12500000000000000, 3.535533905932738641 ) ) ;
#15869=FACE_OUTER_BOUND ( 'NONE', #9052, .T. ) ;
#15870=CARTESIAN_POINT ( 'NONE',  ( 5.000000000000000888, -22.06250000273118772, -2.071067811865475505 ) ) ;
#15877=AXIS2_PLACEMENT_3D ( 'NONE', #4722, #10792, #8458 ) ;
#15887=CIRCLE ( 'NONE', #8928, 5.999999999999991118 ) ;
#15893=CARTESIAN_POINT ( 'NONE',  ( 1.846868145590735200, -26.50000000136559564, -4.458734124999999437 ) ) ;
#15901=CARTESIAN_POINT ( 'NONE',  ( 1.846868145590735200, -22.50000000136559208, -4.458734125000000326 ) ) ;
#15912=DIRECTION ( 'NONE',  ( 1.000000000000000000, 0.000000000000000000, 0.000000000000000000 ) ) ;
#15913=CARTESIAN_POINT ( 'NONE',  ( -3.152801135295367985, -26.81250000136559564, 3.152801135295367096 ) ) ;
#15919=EDGE_LOOP ( 'NONE', ( #11663, #14517, #11689, #15803 ) ) ;
#15920=VERTEX_POINT ( 'NONE', #10630 ) ;
#15921=CYLINDRICAL_SURFACE ( 'NONE', #7995, 5.000000000000000000 ) ;
#15922=CARTESIAN_POINT ( 'NONE',  ( 4.458734124999999437, -23.43750000136559564, 0.000000000000000000 ) ) ;
#15924=EDGE_LOOP ( 'NONE', ( #6595, #10707, #9943, #13931 ) ) ;
#15926=AXIS2_PLACEMENT_3D ( 'NONE', #3646, #6322, #11240 ) ;
#15931=CARTESIAN_POINT ( 'NONE',  ( 4.458734124999999437, -22.75000000136559208, 1.846868145590737864 ) ) ;
#15935=CARTESIAN_POINT ( 'NONE',  ( -9.184850993605147944E-16, -27.37500000273118772, 5.000000000000000000 ) ) ;
#15941=ORIENTED_EDGE ( 'NONE', *, *, #3148, .F. ) ;
#15943=( BOUNDED_CURVE ( )  B_SPLINE_CURVE ( 2, ( #4411, #11902, #2126, #9420, #12957, #5699, #11746, #14195, #5772 ),
 .UNSPECIFIED., .F., .F. ) 
 B_SPLINE_CURVE_WITH_KNOTS ( ( 3, 2, 2, 2, 3 ),
 ( 0.7750000000000000222, 0.7874999999999999778, 0.8000000000000000444, 0.8125000000000001110, 0.8250000000000000666 ),
 .UNSPECIFIED. ) 
 CURVE ( )  GEOMETRIC_REPRESENTATION_ITEM ( )  RATIONAL_B_SPLINE_CURVE ( ( 1.000000000000000000, 0.9238795325112867385, 1.000000000000000000, 0.9238795325112867385, 1.000000000000000000, 0.9238795325112867385, 1.000000000000000000, 0.9238795325112860723, 1.000000000000000666 ) ) 
 REPRESENTATION_ITEM ( '' )  );
#15948=CARTESIAN_POINT ( 'NONE',  ( -5.000000000000000000, -25.62500000273118417, -6.123233995736766282E-16 ) ) ;
#15964=DIRECTION ( 'NONE',  ( -0.000000000000000000, 1.000000000000000000, -0.000000000000000000 ) ) ;
ENDSEC;
END-ISO-10303-21;
